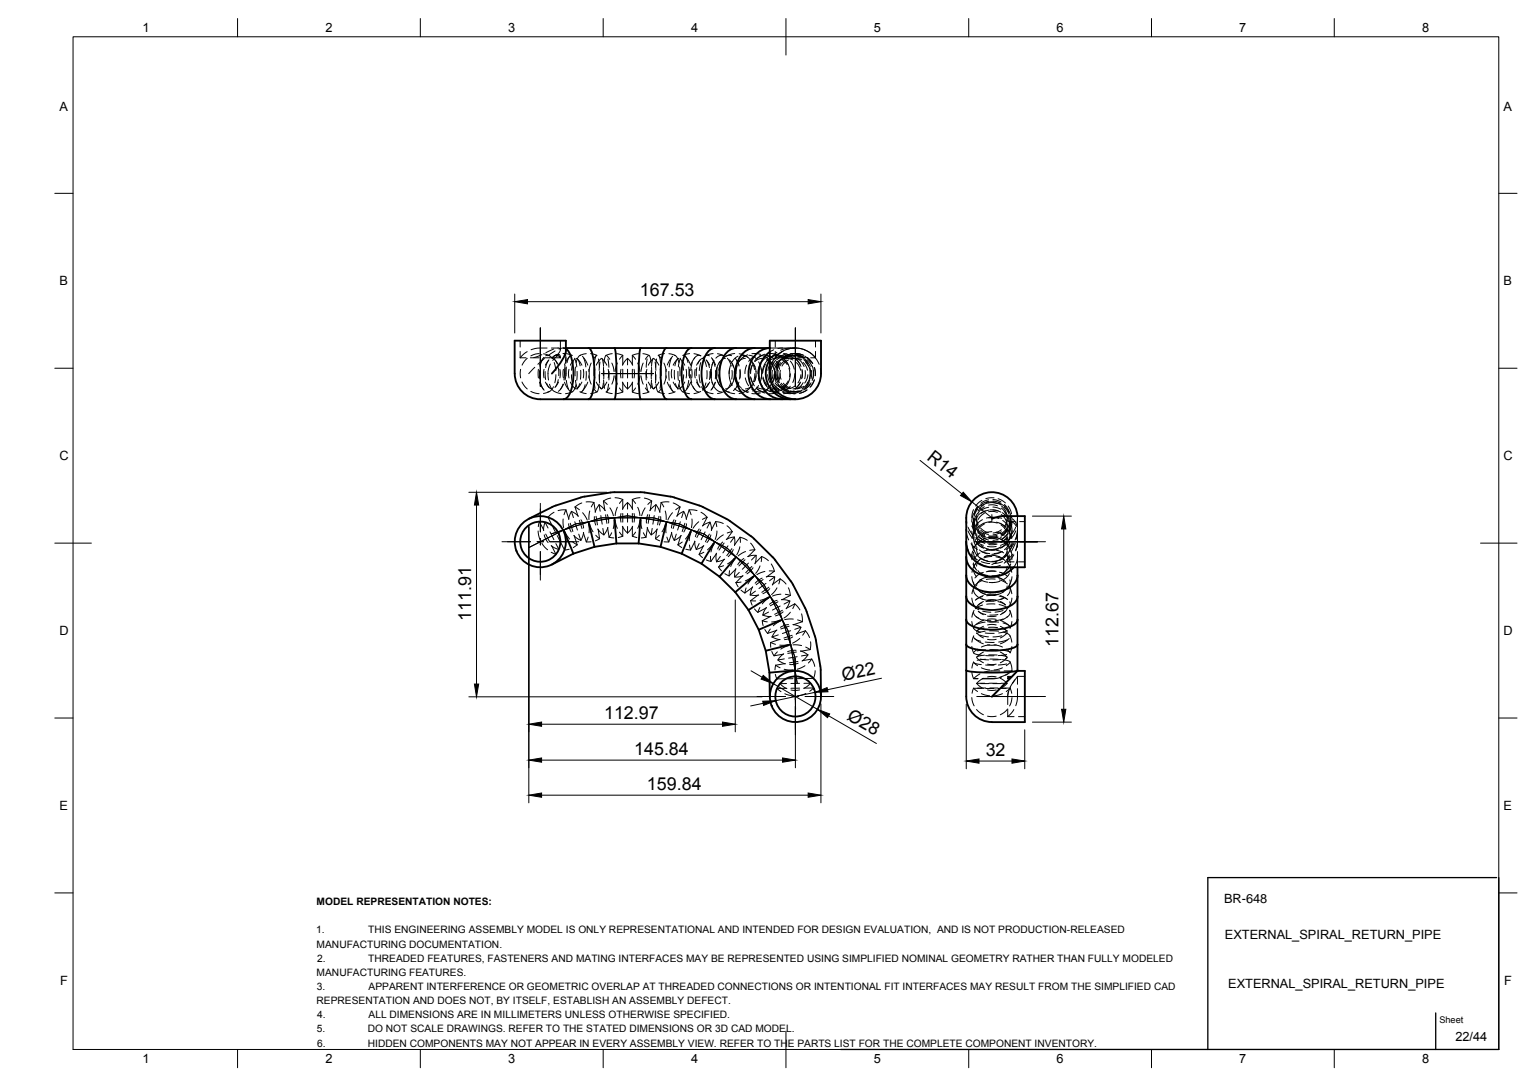
ISO-10303-21;
HEADER;
FILE_DESCRIPTION((''),'2;1');
FILE_NAME('EXTERNAL_SPIRAL_RETURN_PIPE.step','2026-10-01T22:05:39-07:00',(''),(''),'','','');
FILE_SCHEMA (('AUTOMOTIVE_DESIGN { 1 0 10303 214 3 1 1 }'));
ENDSEC;
DATA;
#10=MECHANICAL_DESIGN_GEOMETRIC_PRESENTATION_REPRESENTATION('',(#622),#24628);
#335=ELLIPSE('',#14693,1.97989898732233,1.4) ;
#336=ELLIPSE('',#14696,1.97989898732233,1.4) ;
#337=ELLIPSE('',#14700,1.40426046148572,1.4) ;
#338=ELLIPSE('',#14702,1.40426046148572,1.4) ;
#339=ELLIPSE('',#14708,1.40426046148572,1.4) ;
#340=ELLIPSE('',#14711,1.40426046148572,1.4) ;
#341=ELLIPSE('',#14714,1.40426046148572,1.4) ;
#342=ELLIPSE('',#14719,1.40426046148572,1.4) ;
#343=ELLIPSE('',#14724,1.40426046148572,1.4) ;
#344=ELLIPSE('',#14727,1.40426046148572,1.4) ;
#345=ELLIPSE('',#14730,1.40426046148572,1.4) ;
#346=ELLIPSE('',#14735,1.40426046148572,1.4) ;
#347=ELLIPSE('',#14740,1.40426046148572,1.4) ;
#348=ELLIPSE('',#14743,1.40426046148572,1.4) ;
#349=ELLIPSE('',#14746,1.40426046148572,1.4) ;
#350=ELLIPSE('',#14751,1.40426046148572,1.4) ;
#351=ELLIPSE('',#14756,1.97989898732233,1.4) ;
#352=ELLIPSE('',#14757,1.97989898732233,1.4) ;
#390=SPHERICAL_SURFACE('',#14496,1.1) ;
#391=SPHERICAL_SURFACE('',#14499,1.4) ;
#392=SPHERICAL_SURFACE('',#14501,1.1) ;
#393=SPHERICAL_SURFACE('',#14504,1.1) ;
#394=SPHERICAL_SURFACE('',#14506,1.1) ;
#395=SPHERICAL_SURFACE('',#14510,1.4) ;
#396=SPHERICAL_SURFACE('',#14511,1.4) ;
#397=SPHERICAL_SURFACE('',#14514,1.1) ;
#398=SPHERICAL_SURFACE('',#14517,1.4) ;
#399=SPHERICAL_SURFACE('',#14520,1.1) ;
#400=SPHERICAL_SURFACE('',#14524,1.4) ;
#401=SPHERICAL_SURFACE('',#14526,1.4) ;
#402=SPHERICAL_SURFACE('',#14528,1.1) ;
#403=SPHERICAL_SURFACE('',#14531,1.1) ;
#404=SPHERICAL_SURFACE('',#14533,1.4) ;
#405=SPHERICAL_SURFACE('',#14536,1.1) ;
#406=SPHERICAL_SURFACE('',#14539,1.4) ;
#407=SPHERICAL_SURFACE('',#14541,1.1) ;
#408=SPHERICAL_SURFACE('',#14545,1.4) ;
#409=SPHERICAL_SURFACE('',#14547,1.4) ;
#410=SPHERICAL_SURFACE('',#14549,1.1) ;
#411=SPHERICAL_SURFACE('',#14552,1.1) ;
#412=SPHERICAL_SURFACE('',#14554,1.4) ;
#413=SPHERICAL_SURFACE('',#14557,1.1) ;
#414=SPHERICAL_SURFACE('',#14560,1.4) ;
#415=SPHERICAL_SURFACE('',#14562,1.1) ;
#416=SPHERICAL_SURFACE('',#14566,1.4) ;
#417=SPHERICAL_SURFACE('',#14568,1.4) ;
#418=SPHERICAL_SURFACE('',#14570,1.1) ;
#419=SPHERICAL_SURFACE('',#14573,1.1) ;
#420=SPHERICAL_SURFACE('',#14575,1.4) ;
#421=SPHERICAL_SURFACE('',#14578,1.1) ;
#422=SPHERICAL_SURFACE('',#14581,1.4) ;
#423=SPHERICAL_SURFACE('',#14583,1.1) ;
#424=SPHERICAL_SURFACE('',#14587,1.4) ;
#425=SPHERICAL_SURFACE('',#14589,1.4) ;
#426=SPHERICAL_SURFACE('',#14590,1.1) ;
#427=SPHERICAL_SURFACE('',#14592,1.1) ;
#428=SPHERICAL_SURFACE('',#14593,1.4) ;
#429=SPHERICAL_SURFACE('',#14595,1.1) ;
#430=SPHERICAL_SURFACE('',#14598,1.4) ;
#431=SPHERICAL_SURFACE('',#14599,1.1) ;
#432=SPHERICAL_SURFACE('',#14603,1.4) ;
#433=SPHERICAL_SURFACE('',#14604,1.4) ;
#434=SPHERICAL_SURFACE('',#14605,1.1) ;
#435=SPHERICAL_SURFACE('',#14607,1.1) ;
#436=SPHERICAL_SURFACE('',#14608,1.4) ;
#437=SPHERICAL_SURFACE('',#14610,1.1) ;
#438=SPHERICAL_SURFACE('',#14615,1.4) ;
#439=SPHERICAL_SURFACE('',#14616,1.1) ;
#440=SPHERICAL_SURFACE('',#14622,1.4) ;
#441=SPHERICAL_SURFACE('',#14623,1.4) ;
#442=SPHERICAL_SURFACE('',#14624,1.1) ;
#443=SPHERICAL_SURFACE('',#14626,1.1) ;
#444=SPHERICAL_SURFACE('',#14627,1.4) ;
#445=SPHERICAL_SURFACE('',#14631,1.1) ;
#446=SPHERICAL_SURFACE('',#14632,1.1) ;
#447=SPHERICAL_SURFACE('',#14634,1.1) ;
#448=SPHERICAL_SURFACE('',#14635,1.4) ;
#449=SPHERICAL_SURFACE('',#14638,1.1) ;
#450=SPHERICAL_SURFACE('',#14641,1.4) ;
#451=SPHERICAL_SURFACE('',#14644,1.1) ;
#452=SPHERICAL_SURFACE('',#14650,1.4) ;
#453=SPHERICAL_SURFACE('',#14651,1.4) ;
#454=SPHERICAL_SURFACE('',#14656,1.4) ;
#455=SPHERICAL_SURFACE('',#14661,1.4) ;
#456=SPHERICAL_SURFACE('',#14666,1.4) ;
#457=SPHERICAL_SURFACE('',#14671,1.4) ;
#458=SPHERICAL_SURFACE('',#14676,1.4) ;
#459=SPHERICAL_SURFACE('',#14681,1.4) ;
#460=SPHERICAL_SURFACE('',#14684,1.4) ;
#461=SPHERICAL_SURFACE('',#14763,1.4) ;
#462=SPHERICAL_SURFACE('',#14764,1.4) ;
#463=SPHERICAL_SURFACE('',#14765,1.4) ;
#464=SPHERICAL_SURFACE('',#14766,1.4) ;
#465=SPHERICAL_SURFACE('',#14767,1.4) ;
#466=SPHERICAL_SURFACE('',#14768,1.4) ;
#467=SPHERICAL_SURFACE('',#14769,1.4) ;
#468=SPHERICAL_SURFACE('',#14773,1.4) ;
#469=SPHERICAL_SURFACE('',#14775,1.4) ;
#470=SPHERICAL_SURFACE('',#14776,1.1) ;
#471=SPHERICAL_SURFACE('',#14778,1.1) ;
#472=SPHERICAL_SURFACE('',#14779,1.1) ;
#473=SPHERICAL_SURFACE('',#14781,1.1) ;
#474=SPHERICAL_SURFACE('',#14782,1.1) ;
#475=SPHERICAL_SURFACE('',#14785,1.1) ;
#476=SPHERICAL_SURFACE('',#14787,1.1) ;
#477=SPHERICAL_SURFACE('',#14790,1.1) ;
#478=SPHERICAL_SURFACE('',#14792,1.1) ;
#479=SPHERICAL_SURFACE('',#14795,1.1) ;
#480=SPHERICAL_SURFACE('',#14797,1.1) ;
#481=SPHERICAL_SURFACE('',#14800,1.1) ;
#487=ORIENTED_CLOSED_SHELL('',*,#13133,.F.) ;
#488=ORIENTED_CLOSED_SHELL('',*,#13134,.F.) ;
#489=ORIENTED_CLOSED_SHELL('',*,#13135,.F.) ;
#490=ORIENTED_CLOSED_SHELL('',*,#13136,.F.) ;
#491=ORIENTED_CLOSED_SHELL('',*,#13137,.F.) ;
#492=ORIENTED_CLOSED_SHELL('',*,#13138,.F.) ;
#493=ORIENTED_CLOSED_SHELL('',*,#13139,.F.) ;
#494=ORIENTED_CLOSED_SHELL('',*,#13140,.F.) ;
#495=ORIENTED_CLOSED_SHELL('',*,#13141,.F.) ;
#496=ORIENTED_CLOSED_SHELL('',*,#13142,.F.) ;
#497=ORIENTED_CLOSED_SHELL('',*,#13143,.F.) ;
#498=ORIENTED_CLOSED_SHELL('',*,#13144,.F.) ;
#499=ORIENTED_CLOSED_SHELL('',*,#13145,.F.) ;
#500=ORIENTED_CLOSED_SHELL('',*,#13146,.F.) ;
#501=ORIENTED_CLOSED_SHELL('',*,#13147,.F.) ;
#502=ORIENTED_CLOSED_SHELL('',*,#13148,.F.) ;
#503=ORIENTED_CLOSED_SHELL('',*,#13149,.F.) ;
#504=ORIENTED_CLOSED_SHELL('',*,#13150,.F.) ;
#505=ORIENTED_CLOSED_SHELL('',*,#13151,.F.) ;
#506=ORIENTED_CLOSED_SHELL('',*,#13152,.F.) ;
#507=ORIENTED_CLOSED_SHELL('',*,#13153,.F.) ;
#508=ORIENTED_CLOSED_SHELL('',*,#13154,.F.) ;
#509=ORIENTED_CLOSED_SHELL('',*,#13155,.F.) ;
#510=ORIENTED_CLOSED_SHELL('',*,#13156,.F.) ;
#511=ORIENTED_CLOSED_SHELL('',*,#13157,.F.) ;
#512=ORIENTED_CLOSED_SHELL('',*,#13159,.F.) ;
#513=ORIENTED_CLOSED_SHELL('',*,#13160,.F.) ;
#514=ORIENTED_CLOSED_SHELL('',*,#13161,.F.) ;
#515=ORIENTED_CLOSED_SHELL('',*,#13162,.F.) ;
#516=ORIENTED_CLOSED_SHELL('',*,#13163,.F.) ;
#517=ORIENTED_CLOSED_SHELL('',*,#13164,.F.) ;
#520=BREP_WITH_VOIDS('EXTERNAL_SPIRAL_RETURN_PIPE',#13158,(#487,#488,#489,
#490,#491,#492,#493,#494,#495,#496,#497,#498,#499,#500,#501,#502,#503,#504,
#505,#506,#507,#508,#509,#510,#511,#512,#513,#514,#515,#516,#517)) ;
#538=SHAPE_REPRESENTATION_RELATIONSHIP('SRR','None',#24810,#580) ;
#580=ADVANCED_BREP_SHAPE_REPRESENTATION('',(#520),#24600) ;
#622=STYLED_ITEM('',(#25037),#520) ;
#857=FACE_BOUND('',#4291,.T.) ;
#858=FACE_BOUND('',#4298,.T.) ;
#859=FACE_BOUND('',#4301,.T.) ;
#860=FACE_BOUND('',#4315,.T.) ;
#861=FACE_BOUND('',#4329,.T.) ;
#862=FACE_BOUND('',#4348,.T.) ;
#956=B_SPLINE_CURVE_WITH_KNOTS('',3,(#21637,#21638,#21639,#21640,#21641,
#21642,#21643,#21644,#21645,#21646,#21647,#21648,#21649,#21650),
 .UNSPECIFIED.,.F.,.F.,(4,2,2,2,2,2,4),(1.10605212017019,1.19682866015767,
1.42236457431749,1.64790048847731,1.87343640263713,2.09897231679695,2.18974885678443),
 .UNSPECIFIED.) ;
#957=B_SPLINE_CURVE_WITH_KNOTS('',3,(#21663,#21664,#21665,#21666,#21667,
#21668,#21669,#21670,#21671,#21672,#21673,#21674,#21675,#21676,#21677,#21678,
#21679,#21680,#21681,#21682,#21683,#21684,#21685,#21686,#21687,#21688),
 .UNSPECIFIED.,.F.,.F.,(4,2,2,2,2,2,2,2,2,2,2,2,4),(1.20535125846133,1.58564147586808,
1.96593169327483,2.13946869190595,2.31300569053706,2.5849459608724,2.85688623120774,
3.12882650154308,3.40076677187842,3.57430377050953,3.74784076914065,4.1281309865474,
4.50842120395415),.UNSPECIFIED.) ;
#958=B_SPLINE_CURVE_WITH_KNOTS('',3,(#21860,#21861,#21862,#21863,#21864,
#21865,#21866,#21867,#21868,#21869),.UNSPECIFIED.,.F.,.F.,(4,2,2,2,4),(2.19179053945309,
2.41386787047132,2.73532606912548,3.05678426777964,3.27886159879787),
 .UNSPECIFIED.) ;
#959=B_SPLINE_CURVE_WITH_KNOTS('',3,(#21899,#21900,#21901,#21902,#21903,
#21904,#21905,#21906,#21907,#21908,#21909,#21910,#21911,#21912,#21913,#21914,
#21915,#21916,#21917,#21918,#21919,#21920),.UNSPECIFIED.,.F.,.F.,(4,2,2,
2,2,2,2,2,2,2,4),(1.21055307378235,1.62541412185573,2.04027516992911,2.46215750524915,
2.67309867290916,2.88403984056918,3.0949810082292,3.30592217588921,3.72780451120925,
4.14266555928263,4.557526607356),.UNSPECIFIED.) ;
#960=B_SPLINE_CURVE_WITH_KNOTS('',3,(#21996,#21997,#21998,#21999,#22000,
#22001),.UNSPECIFIED.,.F.,.F.,(4,2,4),(3.13976161696689,3.31479971489035,
3.53911083723209),.UNSPECIFIED.) ;
#961=B_SPLINE_CURVE_WITH_KNOTS('',3,(#22002,#22003,#22004,#22005,#22006,
#22007,#22008,#22009,#22010,#22011,#22012,#22013,#22014,#22015,#22016,#22017,
#22018,#22019,#22020,#22021,#22022,#22023,#22024,#22025),.UNSPECIFIED.,
 .F.,.F.,(4,2,2,2,2,2,2,2,2,2,2,4),(0.,0.224311122341738,0.448622244683475,
0.897244489366951,1.3333999539915,1.55147768630377,1.76955541861604,1.98763315092831,
2.20571088324059,2.64186634786513,3.09048859254861,3.13976161696689),
 .UNSPECIFIED.) ;
#962=B_SPLINE_CURVE_WITH_KNOTS('',3,(#22053,#22054,#22055,#22056,#22057,
#22058,#22059,#22060,#22061,#22062,#22063,#22064,#22065,#22066),
 .UNSPECIFIED.,.F.,.F.,(4,2,2,2,2,2,4),(-3.53911083723208,-3.31479971489035,
-3.09048859254861,-2.64186634786513,-2.20571088324059,-1.98763315092831,
-1.87498686215861),.UNSPECIFIED.) ;
#963=B_SPLINE_CURVE_WITH_KNOTS('',3,(#22068,#22069,#22070,#22071,#22072,
#22073,#22074,#22075,#22076,#22077,#22078,#22079,#22080,#22081,#22082,#22083),
 .UNSPECIFIED.,.F.,.F.,(4,2,2,2,2,2,2,4),(-1.87498686215861,-1.76955541861604,
-1.55147768630377,-1.3333999539915,-0.89724448936695,-0.448622244683476,
-0.224311122341738,0.),.UNSPECIFIED.) ;
#1388=LINE('',#21995,#2224) ;
#1389=LINE('',#22030,#2225) ;
#1390=LINE('',#22043,#2226) ;
#1391=LINE('',#22088,#2227) ;
#1392=LINE('',#22092,#2228) ;
#1393=LINE('',#22096,#2229) ;
#1394=LINE('',#22106,#2230) ;
#1395=LINE('',#22116,#2231) ;
#1396=LINE('',#22120,#2232) ;
#1397=LINE('',#22124,#2233) ;
#1398=LINE('',#22134,#2234) ;
#1399=LINE('',#22144,#2235) ;
#1400=LINE('',#22148,#2236) ;
#1401=LINE('',#22152,#2237) ;
#1402=LINE('',#22162,#2238) ;
#1403=LINE('',#22172,#2239) ;
#1404=LINE('',#22180,#2240) ;
#1405=LINE('',#22194,#2241) ;
#2224=VECTOR('',#17855,1.1) ;
#2225=VECTOR('',#17860,1.4) ;
#2226=VECTOR('',#17875,1.4) ;
#2227=VECTOR('',#17892,1.4) ;
#2228=VECTOR('',#17899,1.4) ;
#2229=VECTOR('',#17904,1.4) ;
#2230=VECTOR('',#17915,1.4) ;
#2231=VECTOR('',#17928,1.4) ;
#2232=VECTOR('',#17935,1.4) ;
#2233=VECTOR('',#17940,1.4) ;
#2234=VECTOR('',#17951,1.4) ;
#2235=VECTOR('',#17964,1.4) ;
#2236=VECTOR('',#17971,1.4) ;
#2237=VECTOR('',#17976,1.4) ;
#2238=VECTOR('',#17987,1.4) ;
#2239=VECTOR('',#18000,1.4) ;
#2240=VECTOR('',#18011,1.4) ;
#2241=VECTOR('',#18036,1.1) ;
#2844=CYLINDRICAL_SURFACE('',#14508,1.1) ;
#2845=CYLINDRICAL_SURFACE('',#14519,1.4) ;
#2846=CYLINDRICAL_SURFACE('',#14630,1.1) ;
#2847=CYLINDRICAL_SURFACE('',#14649,1.4) ;
#2848=CYLINDRICAL_SURFACE('',#14689,1.1) ;
#2849=CYLINDRICAL_SURFACE('',#14691,1.4) ;
#2850=CYLINDRICAL_SURFACE('',#14699,1.4) ;
#2851=CYLINDRICAL_SURFACE('',#14704,1.4) ;
#2852=CYLINDRICAL_SURFACE('',#14706,1.4) ;
#2853=CYLINDRICAL_SURFACE('',#14710,1.4) ;
#2854=CYLINDRICAL_SURFACE('',#14712,1.4) ;
#2855=CYLINDRICAL_SURFACE('',#14716,1.4) ;
#2856=CYLINDRICAL_SURFACE('',#14722,1.4) ;
#2857=CYLINDRICAL_SURFACE('',#14726,1.4) ;
#2858=CYLINDRICAL_SURFACE('',#14728,1.4) ;
#2859=CYLINDRICAL_SURFACE('',#14732,1.4) ;
#2860=CYLINDRICAL_SURFACE('',#14738,1.4) ;
#2861=CYLINDRICAL_SURFACE('',#14742,1.4) ;
#2862=CYLINDRICAL_SURFACE('',#14744,1.4) ;
#2863=CYLINDRICAL_SURFACE('',#14748,1.4) ;
#2864=CYLINDRICAL_SURFACE('',#14754,1.4) ;
#2865=CYLINDRICAL_SURFACE('',#14759,1.4) ;
#2866=CYLINDRICAL_SURFACE('',#14760,1.4) ;
#2867=CYLINDRICAL_SURFACE('',#14771,1.1) ;
#3309=FACE_OUTER_BOUND('',#4247,.T.) ;
#3310=FACE_OUTER_BOUND('',#4248,.T.) ;
#3311=FACE_OUTER_BOUND('',#4249,.T.) ;
#3312=FACE_OUTER_BOUND('',#4250,.T.) ;
#3313=FACE_OUTER_BOUND('',#4251,.T.) ;
#3314=FACE_OUTER_BOUND('',#4252,.T.) ;
#3315=FACE_OUTER_BOUND('',#4253,.T.) ;
#3316=FACE_OUTER_BOUND('',#4254,.T.) ;
#3317=FACE_OUTER_BOUND('',#4255,.T.) ;
#3318=FACE_OUTER_BOUND('',#4256,.T.) ;
#3319=FACE_OUTER_BOUND('',#4257,.T.) ;
#3320=FACE_OUTER_BOUND('',#4258,.T.) ;
#3321=FACE_OUTER_BOUND('',#4259,.T.) ;
#3322=FACE_OUTER_BOUND('',#4260,.T.) ;
#3323=FACE_OUTER_BOUND('',#4261,.T.) ;
#3324=FACE_OUTER_BOUND('',#4262,.T.) ;
#3325=FACE_OUTER_BOUND('',#4263,.T.) ;
#3326=FACE_OUTER_BOUND('',#4264,.T.) ;
#3327=FACE_OUTER_BOUND('',#4265,.T.) ;
#3328=FACE_OUTER_BOUND('',#4266,.T.) ;
#3329=FACE_OUTER_BOUND('',#4267,.T.) ;
#3330=FACE_OUTER_BOUND('',#4268,.T.) ;
#3331=FACE_OUTER_BOUND('',#4269,.T.) ;
#3332=FACE_OUTER_BOUND('',#4270,.T.) ;
#3333=FACE_OUTER_BOUND('',#4271,.T.) ;
#3334=FACE_OUTER_BOUND('',#4272,.T.) ;
#3335=FACE_OUTER_BOUND('',#4273,.T.) ;
#3336=FACE_OUTER_BOUND('',#4274,.T.) ;
#3337=FACE_OUTER_BOUND('',#4275,.T.) ;
#3338=FACE_OUTER_BOUND('',#4276,.T.) ;
#3339=FACE_OUTER_BOUND('',#4277,.T.) ;
#3340=FACE_OUTER_BOUND('',#4278,.T.) ;
#3341=FACE_OUTER_BOUND('',#4279,.T.) ;
#3342=FACE_OUTER_BOUND('',#4280,.T.) ;
#3343=FACE_OUTER_BOUND('',#4281,.T.) ;
#3344=FACE_OUTER_BOUND('',#4282,.T.) ;
#3345=FACE_OUTER_BOUND('',#4283,.T.) ;
#3346=FACE_OUTER_BOUND('',#4284,.T.) ;
#3347=FACE_OUTER_BOUND('',#4285,.T.) ;
#3348=FACE_OUTER_BOUND('',#4286,.T.) ;
#3349=FACE_OUTER_BOUND('',#4287,.T.) ;
#3350=FACE_OUTER_BOUND('',#4288,.T.) ;
#3351=FACE_OUTER_BOUND('',#4289,.T.) ;
#3352=FACE_OUTER_BOUND('',#4290,.T.) ;
#3353=FACE_OUTER_BOUND('',#4292,.T.) ;
#3354=FACE_OUTER_BOUND('',#4293,.T.) ;
#3355=FACE_OUTER_BOUND('',#4294,.T.) ;
#3356=FACE_OUTER_BOUND('',#4295,.T.) ;
#3357=FACE_OUTER_BOUND('',#4296,.T.) ;
#3358=FACE_OUTER_BOUND('',#4297,.T.) ;
#3359=FACE_OUTER_BOUND('',#4299,.T.) ;
#3360=FACE_OUTER_BOUND('',#4300,.T.) ;
#3361=FACE_OUTER_BOUND('',#4302,.T.) ;
#3362=FACE_OUTER_BOUND('',#4303,.T.) ;
#3363=FACE_OUTER_BOUND('',#4304,.T.) ;
#3364=FACE_OUTER_BOUND('',#4305,.T.) ;
#3365=FACE_OUTER_BOUND('',#4306,.T.) ;
#3366=FACE_OUTER_BOUND('',#4307,.T.) ;
#3367=FACE_OUTER_BOUND('',#4308,.T.) ;
#3368=FACE_OUTER_BOUND('',#4309,.T.) ;
#3369=FACE_OUTER_BOUND('',#4310,.T.) ;
#3370=FACE_OUTER_BOUND('',#4311,.T.) ;
#3371=FACE_OUTER_BOUND('',#4312,.T.) ;
#3372=FACE_OUTER_BOUND('',#4313,.T.) ;
#3373=FACE_OUTER_BOUND('',#4314,.T.) ;
#3374=FACE_OUTER_BOUND('',#4316,.T.) ;
#3375=FACE_OUTER_BOUND('',#4317,.T.) ;
#3376=FACE_OUTER_BOUND('',#4318,.T.) ;
#3377=FACE_OUTER_BOUND('',#4319,.T.) ;
#3378=FACE_OUTER_BOUND('',#4320,.T.) ;
#3379=FACE_OUTER_BOUND('',#4321,.T.) ;
#3380=FACE_OUTER_BOUND('',#4322,.T.) ;
#3381=FACE_OUTER_BOUND('',#4323,.T.) ;
#3382=FACE_OUTER_BOUND('',#4324,.T.) ;
#3383=FACE_OUTER_BOUND('',#4325,.T.) ;
#3384=FACE_OUTER_BOUND('',#4326,.T.) ;
#3385=FACE_OUTER_BOUND('',#4327,.T.) ;
#3386=FACE_OUTER_BOUND('',#4328,.T.) ;
#3387=FACE_OUTER_BOUND('',#4330,.T.) ;
#3388=FACE_OUTER_BOUND('',#4331,.T.) ;
#3389=FACE_OUTER_BOUND('',#4332,.T.) ;
#3390=FACE_OUTER_BOUND('',#4333,.T.) ;
#3391=FACE_OUTER_BOUND('',#4334,.T.) ;
#3392=FACE_OUTER_BOUND('',#4335,.T.) ;
#3393=FACE_OUTER_BOUND('',#4336,.T.) ;
#3394=FACE_OUTER_BOUND('',#4337,.T.) ;
#3395=FACE_OUTER_BOUND('',#4338,.T.) ;
#3396=FACE_OUTER_BOUND('',#4339,.T.) ;
#3397=FACE_OUTER_BOUND('',#4340,.T.) ;
#3398=FACE_OUTER_BOUND('',#4341,.T.) ;
#3399=FACE_OUTER_BOUND('',#4342,.T.) ;
#3400=FACE_OUTER_BOUND('',#4343,.T.) ;
#3401=FACE_OUTER_BOUND('',#4344,.T.) ;
#3402=FACE_OUTER_BOUND('',#4345,.T.) ;
#3403=FACE_OUTER_BOUND('',#4346,.T.) ;
#3404=FACE_OUTER_BOUND('',#4347,.T.) ;
#3405=FACE_OUTER_BOUND('',#4349,.T.) ;
#3406=FACE_OUTER_BOUND('',#4350,.T.) ;
#3407=FACE_OUTER_BOUND('',#4351,.T.) ;
#3408=FACE_OUTER_BOUND('',#4352,.T.) ;
#3409=FACE_OUTER_BOUND('',#4353,.T.) ;
#3410=FACE_OUTER_BOUND('',#4354,.T.) ;
#3411=FACE_OUTER_BOUND('',#4355,.T.) ;
#3412=FACE_OUTER_BOUND('',#4356,.T.) ;
#3413=FACE_OUTER_BOUND('',#4357,.T.) ;
#3414=FACE_OUTER_BOUND('',#4358,.T.) ;
#3415=FACE_OUTER_BOUND('',#4359,.T.) ;
#3416=FACE_OUTER_BOUND('',#4360,.T.) ;
#3417=FACE_OUTER_BOUND('',#4361,.T.) ;
#3418=FACE_OUTER_BOUND('',#4362,.T.) ;
#3419=FACE_OUTER_BOUND('',#4363,.T.) ;
#3420=FACE_OUTER_BOUND('',#4364,.T.) ;
#3421=FACE_OUTER_BOUND('',#4365,.T.) ;
#3422=FACE_OUTER_BOUND('',#4366,.T.) ;
#3423=FACE_OUTER_BOUND('',#4367,.T.) ;
#3424=FACE_OUTER_BOUND('',#4368,.T.) ;
#3425=FACE_OUTER_BOUND('',#4369,.T.) ;
#3426=FACE_OUTER_BOUND('',#4370,.T.) ;
#4247=EDGE_LOOP('',(#10205,#10206,#10207)) ;
#4248=EDGE_LOOP('',(#10208,#10209,#10210)) ;
#4249=EDGE_LOOP('',(#10211,#10212,#10213)) ;
#4250=EDGE_LOOP('',(#10214,#10215,#10216)) ;
#4251=EDGE_LOOP('',(#10217,#10218)) ;
#4252=EDGE_LOOP('',(#10219,#10220)) ;
#4253=EDGE_LOOP('',(#10221,#10222)) ;
#4254=EDGE_LOOP('',(#10223,#10224,#10225)) ;
#4255=EDGE_LOOP('',(#10226,#10227,#10228,#10229,#10230)) ;
#4256=EDGE_LOOP('',(#10231,#10232)) ;
#4257=EDGE_LOOP('',(#10233,#10234)) ;
#4258=EDGE_LOOP('',(#10235,#10236,#10237,#10238)) ;
#4259=EDGE_LOOP('',(#10239,#10240,#10241)) ;
#4260=EDGE_LOOP('',(#10242,#10243,#10244)) ;
#4261=EDGE_LOOP('',(#10245,#10246,#10247)) ;
#4262=EDGE_LOOP('',(#10248,#10249,#10250)) ;
#4263=EDGE_LOOP('',(#10251,#10252,#10253)) ;
#4264=EDGE_LOOP('',(#10254,#10255,#10256,#10257)) ;
#4265=EDGE_LOOP('',(#10258,#10259,#10260)) ;
#4266=EDGE_LOOP('',(#10261,#10262,#10263,#10264)) ;
#4267=EDGE_LOOP('',(#10265,#10266,#10267)) ;
#4268=EDGE_LOOP('',(#10268,#10269,#10270)) ;
#4269=EDGE_LOOP('',(#10271,#10272,#10273)) ;
#4270=EDGE_LOOP('',(#10274,#10275,#10276)) ;
#4271=EDGE_LOOP('',(#10277,#10278,#10279)) ;
#4272=EDGE_LOOP('',(#10280,#10281,#10282,#10283)) ;
#4273=EDGE_LOOP('',(#10284,#10285,#10286)) ;
#4274=EDGE_LOOP('',(#10287,#10288,#10289,#10290)) ;
#4275=EDGE_LOOP('',(#10291,#10292,#10293)) ;
#4276=EDGE_LOOP('',(#10294,#10295,#10296)) ;
#4277=EDGE_LOOP('',(#10297,#10298,#10299)) ;
#4278=EDGE_LOOP('',(#10300,#10301,#10302)) ;
#4279=EDGE_LOOP('',(#10303,#10304,#10305)) ;
#4280=EDGE_LOOP('',(#10306,#10307,#10308,#10309)) ;
#4281=EDGE_LOOP('',(#10310,#10311,#10312)) ;
#4282=EDGE_LOOP('',(#10313,#10314,#10315,#10316)) ;
#4283=EDGE_LOOP('',(#10317,#10318,#10319)) ;
#4284=EDGE_LOOP('',(#10320)) ;
#4285=EDGE_LOOP('',(#10321)) ;
#4286=EDGE_LOOP('',(#10322)) ;
#4287=EDGE_LOOP('',(#10323)) ;
#4288=EDGE_LOOP('',(#10324,#10325,#10326,#10327)) ;
#4289=EDGE_LOOP('',(#10328)) ;
#4290=EDGE_LOOP('',(#10329,#10330,#10331)) ;
#4291=EDGE_LOOP('',(#10332)) ;
#4292=EDGE_LOOP('',(#10333)) ;
#4293=EDGE_LOOP('',(#10334)) ;
#4294=EDGE_LOOP('',(#10335)) ;
#4295=EDGE_LOOP('',(#10336)) ;
#4296=EDGE_LOOP('',(#10337)) ;
#4297=EDGE_LOOP('',(#10338,#10339,#10340,#10341,#10342,#10343)) ;
#4298=EDGE_LOOP('',(#10344)) ;
#4299=EDGE_LOOP('',(#10345,#10346)) ;
#4300=EDGE_LOOP('',(#10347,#10348,#10349,#10350,#10351,#10352)) ;
#4301=EDGE_LOOP('',(#10353)) ;
#4302=EDGE_LOOP('',(#10354,#10355)) ;
#4303=EDGE_LOOP('',(#10356)) ;
#4304=EDGE_LOOP('',(#10357)) ;
#4305=EDGE_LOOP('',(#10358)) ;
#4306=EDGE_LOOP('',(#10359,#10360)) ;
#4307=EDGE_LOOP('',(#10361,#10362)) ;
#4308=EDGE_LOOP('',(#10363,#10364)) ;
#4309=EDGE_LOOP('',(#10365)) ;
#4310=EDGE_LOOP('',(#10366)) ;
#4311=EDGE_LOOP('',(#10367,#10368)) ;
#4312=EDGE_LOOP('',(#10369,#10370,#10371,#10372,#10373,#10374)) ;
#4313=EDGE_LOOP('',(#10375,#10376)) ;
#4314=EDGE_LOOP('',(#10377,#10378,#10379,#10380,#10381,#10382)) ;
#4315=EDGE_LOOP('',(#10383,#10384)) ;
#4316=EDGE_LOOP('',(#10385,#10386)) ;
#4317=EDGE_LOOP('',(#10387,#10388)) ;
#4318=EDGE_LOOP('',(#10389,#10390,#10391,#10392)) ;
#4319=EDGE_LOOP('',(#10393,#10394,#10395,#10396)) ;
#4320=EDGE_LOOP('',(#10397,#10398,#10399,#10400)) ;
#4321=EDGE_LOOP('',(#10401,#10402,#10403,#10404)) ;
#4322=EDGE_LOOP('',(#10405,#10406,#10407,#10408)) ;
#4323=EDGE_LOOP('',(#10409,#10410,#10411,#10412)) ;
#4324=EDGE_LOOP('',(#10413,#10414)) ;
#4325=EDGE_LOOP('',(#10415,#10416,#10417,#10418,#10419)) ;
#4326=EDGE_LOOP('',(#10420,#10421,#10422,#10423,#10424,#10425)) ;
#4327=EDGE_LOOP('',(#10426,#10427,#10428,#10429,#10430,#10431,#10432)) ;
#4328=EDGE_LOOP('',(#10433)) ;
#4329=EDGE_LOOP('',(#10434)) ;
#4330=EDGE_LOOP('',(#10435,#10436,#10437,#10438,#10439,#10440,#10441,#10442)) ;
#4331=EDGE_LOOP('',(#10443,#10444,#10445)) ;
#4332=EDGE_LOOP('',(#10446,#10447,#10448,#10449,#10450,#10451,#10452,#10453,
#10454)) ;
#4333=EDGE_LOOP('',(#10455,#10456,#10457,#10458,#10459,#10460,#10461,#10462)) ;
#4334=EDGE_LOOP('',(#10463,#10464,#10465,#10466,#10467,#10468,#10469,#10470)) ;
#4335=EDGE_LOOP('',(#10471,#10472,#10473,#10474,#10475,#10476,#10477,#10478)) ;
#4336=EDGE_LOOP('',(#10479,#10480,#10481,#10482,#10483,#10484,#10485,#10486)) ;
#4337=EDGE_LOOP('',(#10487,#10488,#10489,#10490,#10491,#10492,#10493,#10494)) ;
#4338=EDGE_LOOP('',(#10495,#10496,#10497,#10498,#10499,#10500,#10501,#10502)) ;
#4339=EDGE_LOOP('',(#10503,#10504,#10505,#10506,#10507,#10508,#10509,#10510)) ;
#4340=EDGE_LOOP('',(#10511,#10512,#10513,#10514,#10515,#10516,#10517,#10518)) ;
#4341=EDGE_LOOP('',(#10519,#10520,#10521,#10522,#10523,#10524,#10525,#10526)) ;
#4342=EDGE_LOOP('',(#10527,#10528,#10529,#10530,#10531,#10532,#10533,#10534)) ;
#4343=EDGE_LOOP('',(#10535,#10536,#10537,#10538,#10539,#10540,#10541,#10542)) ;
#4344=EDGE_LOOP('',(#10543,#10544,#10545,#10546,#10547,#10548,#10549,#10550,
#10551)) ;
#4345=EDGE_LOOP('',(#10552,#10553,#10554)) ;
#4346=EDGE_LOOP('',(#10555,#10556,#10557,#10558,#10559,#10560)) ;
#4347=EDGE_LOOP('',(#10561)) ;
#4348=EDGE_LOOP('',(#10562)) ;
#4349=EDGE_LOOP('',(#10563,#10564,#10565,#10566)) ;
#4350=EDGE_LOOP('',(#10567,#10568,#10569,#10570)) ;
#4351=EDGE_LOOP('',(#10571,#10572,#10573,#10574)) ;
#4352=EDGE_LOOP('',(#10575,#10576,#10577,#10578)) ;
#4353=EDGE_LOOP('',(#10579,#10580,#10581,#10582)) ;
#4354=EDGE_LOOP('',(#10583,#10584,#10585,#10586)) ;
#4355=EDGE_LOOP('',(#10587,#10588,#10589,#10590,#10591)) ;
#4356=EDGE_LOOP('',(#10592,#10593,#10594,#10595,#10596,#10597)) ;
#4357=EDGE_LOOP('',(#10598,#10599,#10600,#10601,#10602)) ;
#4358=EDGE_LOOP('',(#10603,#10604)) ;
#4359=EDGE_LOOP('',(#10605)) ;
#4360=EDGE_LOOP('',(#10606)) ;
#4361=EDGE_LOOP('',(#10607)) ;
#4362=EDGE_LOOP('',(#10608)) ;
#4363=EDGE_LOOP('',(#10609,#10610,#10611)) ;
#4364=EDGE_LOOP('',(#10612,#10613,#10614)) ;
#4365=EDGE_LOOP('',(#10615,#10616,#10617)) ;
#4366=EDGE_LOOP('',(#10618,#10619,#10620)) ;
#4367=EDGE_LOOP('',(#10621,#10622,#10623)) ;
#4368=EDGE_LOOP('',(#10624,#10625,#10626)) ;
#4369=EDGE_LOOP('',(#10627,#10628,#10629)) ;
#4370=EDGE_LOOP('',(#10630,#10631,#10632)) ;
#5160=CIRCLE('',#14497,1.00181590545205) ;
#5161=CIRCLE('',#14498,1.1) ;
#5162=CIRCLE('',#14500,1.4) ;
#5163=CIRCLE('',#14502,0.834979872033575) ;
#5164=CIRCLE('',#14503,1.1) ;
#5165=CIRCLE('',#14505,1.1) ;
#5166=CIRCLE('',#14507,1.00181590545205) ;
#5167=CIRCLE('',#14509,1.1) ;
#5168=CIRCLE('',#14512,1.00181590545205) ;
#5169=CIRCLE('',#14513,1.4) ;
#5170=CIRCLE('',#14515,1.1) ;
#5171=CIRCLE('',#14516,1.00181590545205) ;
#5172=CIRCLE('',#14518,1.4) ;
#5173=CIRCLE('',#14521,1.00181590545205) ;
#5174=CIRCLE('',#14522,1.1) ;
#5175=CIRCLE('',#14523,1.00181590545205) ;
#5176=CIRCLE('',#14525,1.4) ;
#5177=CIRCLE('',#14527,1.4) ;
#5178=CIRCLE('',#14529,0.834979872033575) ;
#5179=CIRCLE('',#14530,1.1) ;
#5180=CIRCLE('',#14532,1.1) ;
#5181=CIRCLE('',#14534,1.00181590545205) ;
#5182=CIRCLE('',#14535,1.4) ;
#5183=CIRCLE('',#14537,1.1) ;
#5184=CIRCLE('',#14538,1.00181590545205) ;
#5185=CIRCLE('',#14540,1.4) ;
#5186=CIRCLE('',#14542,1.00181590545205) ;
#5187=CIRCLE('',#14543,1.1) ;
#5188=CIRCLE('',#14544,1.00181590545205) ;
#5189=CIRCLE('',#14546,1.4) ;
#5190=CIRCLE('',#14548,1.4) ;
#5191=CIRCLE('',#14550,0.834979872033577) ;
#5192=CIRCLE('',#14551,1.1) ;
#5193=CIRCLE('',#14553,1.1) ;
#5194=CIRCLE('',#14555,1.00181590545205) ;
#5195=CIRCLE('',#14556,1.4) ;
#5196=CIRCLE('',#14558,1.1) ;
#5197=CIRCLE('',#14559,1.00181590545205) ;
#5198=CIRCLE('',#14561,1.4) ;
#5199=CIRCLE('',#14563,1.00181590545205) ;
#5200=CIRCLE('',#14564,1.1) ;
#5201=CIRCLE('',#14565,1.00181590545205) ;
#5202=CIRCLE('',#14567,1.4) ;
#5203=CIRCLE('',#14569,1.4) ;
#5204=CIRCLE('',#14571,0.834979872033573) ;
#5205=CIRCLE('',#14572,1.1) ;
#5206=CIRCLE('',#14574,1.1) ;
#5207=CIRCLE('',#14576,1.00181590545205) ;
#5208=CIRCLE('',#14577,1.4) ;
#5209=CIRCLE('',#14579,1.1) ;
#5210=CIRCLE('',#14580,1.00181590545205) ;
#5211=CIRCLE('',#14582,1.4) ;
#5212=CIRCLE('',#14584,1.00181590545205) ;
#5213=CIRCLE('',#14585,1.1) ;
#5214=CIRCLE('',#14586,1.00181590545205) ;
#5215=CIRCLE('',#14588,1.4) ;
#5216=CIRCLE('',#14591,0.834979872033577) ;
#5217=CIRCLE('',#14594,1.00181590545205) ;
#5218=CIRCLE('',#14596,1.1) ;
#5219=CIRCLE('',#14597,1.00181590545205) ;
#5220=CIRCLE('',#14600,1.00181590545205) ;
#5221=CIRCLE('',#14601,1.1) ;
#5222=CIRCLE('',#14602,1.00181590545205) ;
#5223=CIRCLE('',#14606,0.834979872033575) ;
#5224=CIRCLE('',#14609,1.00181590545205) ;
#5225=CIRCLE('',#14611,1.00181590545205) ;
#5226=CIRCLE('',#14612,1.1) ;
#5227=CIRCLE('',#14613,1.00181590545205) ;
#5228=CIRCLE('',#14614,1.1) ;
#5229=CIRCLE('',#14617,1.00181590545205) ;
#5230=CIRCLE('',#14618,1.1) ;
#5231=CIRCLE('',#14619,1.00181590545205) ;
#5232=CIRCLE('',#14620,1.1) ;
#5233=CIRCLE('',#14621,1.00181590545205) ;
#5234=CIRCLE('',#14625,0.834979872033575) ;
#5235=CIRCLE('',#14628,1.00181590545205) ;
#5236=CIRCLE('',#14629,1.1) ;
#5237=CIRCLE('',#14633,0.834979872033575) ;
#5238=CIRCLE('',#14636,1.00181590545205) ;
#5239=CIRCLE('',#14637,1.00181590545205) ;
#5240=CIRCLE('',#14639,1.1) ;
#5241=CIRCLE('',#14640,1.1) ;
#5242=CIRCLE('',#14642,1.00181590545205) ;
#5243=CIRCLE('',#14643,1.4) ;
#5244=CIRCLE('',#14645,1.00181590545205) ;
#5245=CIRCLE('',#14646,1.1) ;
#5246=CIRCLE('',#14647,1.00181590545205) ;
#5247=CIRCLE('',#14648,1.1) ;
#5248=CIRCLE('',#14652,1.4) ;
#5249=CIRCLE('',#14653,1.4) ;
#5250=CIRCLE('',#14654,1.4) ;
#5251=CIRCLE('',#14655,1.4) ;
#5252=CIRCLE('',#14657,1.4) ;
#5253=CIRCLE('',#14658,1.4) ;
#5254=CIRCLE('',#14659,1.4) ;
#5255=CIRCLE('',#14660,1.4) ;
#5256=CIRCLE('',#14662,1.4) ;
#5257=CIRCLE('',#14663,1.4) ;
#5258=CIRCLE('',#14664,1.4) ;
#5259=CIRCLE('',#14665,1.4) ;
#5260=CIRCLE('',#14667,1.4) ;
#5261=CIRCLE('',#14668,1.4) ;
#5262=CIRCLE('',#14669,1.4) ;
#5263=CIRCLE('',#14670,1.4) ;
#5264=CIRCLE('',#14672,1.4) ;
#5265=CIRCLE('',#14673,1.4) ;
#5266=CIRCLE('',#14674,1.4) ;
#5267=CIRCLE('',#14675,1.4) ;
#5268=CIRCLE('',#14677,1.4) ;
#5269=CIRCLE('',#14678,1.4) ;
#5270=CIRCLE('',#14679,1.4) ;
#5271=CIRCLE('',#14680,1.4) ;
#5272=CIRCLE('',#14682,1.4) ;
#5273=CIRCLE('',#14683,1.1) ;
#5274=CIRCLE('',#14685,1.4) ;
#5275=CIRCLE('',#14686,1.4) ;
#5276=CIRCLE('',#14687,1.4) ;
#5277=CIRCLE('',#14688,1.4) ;
#5278=CIRCLE('',#14690,1.1) ;
#5279=CIRCLE('',#14692,1.4) ;
#5280=CIRCLE('',#14694,1.4) ;
#5281=CIRCLE('',#14695,1.4) ;
#5282=CIRCLE('',#14698,1.1) ;
#5283=CIRCLE('',#14701,1.4) ;
#5284=CIRCLE('',#14703,1.4) ;
#5285=CIRCLE('',#14705,1.4) ;
#5286=CIRCLE('',#14707,1.4) ;
#5287=CIRCLE('',#14709,1.4) ;
#5288=CIRCLE('',#14713,1.4) ;
#5289=CIRCLE('',#14715,1.4) ;
#5290=CIRCLE('',#14717,1.4) ;
#5291=CIRCLE('',#14718,1.4) ;
#5292=CIRCLE('',#14720,1.4) ;
#5293=CIRCLE('',#14721,1.4) ;
#5294=CIRCLE('',#14723,1.4) ;
#5295=CIRCLE('',#14725,1.4) ;
#5296=CIRCLE('',#14729,1.4) ;
#5297=CIRCLE('',#14731,1.4) ;
#5298=CIRCLE('',#14733,1.4) ;
#5299=CIRCLE('',#14734,1.4) ;
#5300=CIRCLE('',#14736,1.4) ;
#5301=CIRCLE('',#14737,1.4) ;
#5302=CIRCLE('',#14739,1.4) ;
#5303=CIRCLE('',#14741,1.4) ;
#5304=CIRCLE('',#14745,1.4) ;
#5305=CIRCLE('',#14747,1.4) ;
#5306=CIRCLE('',#14749,1.4) ;
#5307=CIRCLE('',#14750,1.4) ;
#5308=CIRCLE('',#14752,1.4) ;
#5309=CIRCLE('',#14753,1.4) ;
#5310=CIRCLE('',#14755,1.4) ;
#5311=CIRCLE('',#14758,1.4) ;
#5312=CIRCLE('',#14761,1.4) ;
#5313=CIRCLE('',#14770,1.4) ;
#5314=CIRCLE('',#14772,1.1) ;
#5315=CIRCLE('',#14774,1.4) ;
#5316=CIRCLE('',#14777,0.834979872033575) ;
#5317=CIRCLE('',#14780,0.834979872033575) ;
#5318=CIRCLE('',#14783,0.834979872033573) ;
#5319=CIRCLE('',#14784,1.1) ;
#5320=CIRCLE('',#14786,1.1) ;
#5321=CIRCLE('',#14788,0.834979872033575) ;
#5322=CIRCLE('',#14789,1.1) ;
#5323=CIRCLE('',#14791,1.1) ;
#5324=CIRCLE('',#14793,0.834979872033573) ;
#5325=CIRCLE('',#14794,1.1) ;
#5326=CIRCLE('',#14796,1.1) ;
#5327=CIRCLE('',#14798,0.834979872033575) ;
#5328=CIRCLE('',#14799,1.1) ;
#5329=CIRCLE('',#14801,1.1) ;
#6114=VERTEX_POINT('',#21618) ;
#6115=VERTEX_POINT('',#21620) ;
#6116=VERTEX_POINT('',#21623) ;
#6117=VERTEX_POINT('',#21626) ;
#6118=VERTEX_POINT('',#21628) ;
#6119=VERTEX_POINT('',#21631) ;
#6120=VERTEX_POINT('',#21634) ;
#6121=VERTEX_POINT('',#21635) ;
#6122=VERTEX_POINT('',#21655) ;
#6123=VERTEX_POINT('',#21657) ;
#6124=VERTEX_POINT('',#21660) ;
#6125=VERTEX_POINT('',#21662) ;
#6126=VERTEX_POINT('',#21694) ;
#6127=VERTEX_POINT('',#21696) ;
#6128=VERTEX_POINT('',#21700) ;
#6129=VERTEX_POINT('',#21703) ;
#6130=VERTEX_POINT('',#21706) ;
#6131=VERTEX_POINT('',#21708) ;
#6132=VERTEX_POINT('',#21711) ;
#6133=VERTEX_POINT('',#21714) ;
#6134=VERTEX_POINT('',#21716) ;
#6135=VERTEX_POINT('',#21719) ;
#6136=VERTEX_POINT('',#21723) ;
#6137=VERTEX_POINT('',#21726) ;
#6138=VERTEX_POINT('',#21728) ;
#6139=VERTEX_POINT('',#21732) ;
#6140=VERTEX_POINT('',#21735) ;
#6141=VERTEX_POINT('',#21738) ;
#6142=VERTEX_POINT('',#21740) ;
#6143=VERTEX_POINT('',#21743) ;
#6144=VERTEX_POINT('',#21746) ;
#6145=VERTEX_POINT('',#21748) ;
#6146=VERTEX_POINT('',#21751) ;
#6147=VERTEX_POINT('',#21755) ;
#6148=VERTEX_POINT('',#21758) ;
#6149=VERTEX_POINT('',#21760) ;
#6150=VERTEX_POINT('',#21764) ;
#6151=VERTEX_POINT('',#21767) ;
#6152=VERTEX_POINT('',#21770) ;
#6153=VERTEX_POINT('',#21772) ;
#6154=VERTEX_POINT('',#21775) ;
#6155=VERTEX_POINT('',#21778) ;
#6156=VERTEX_POINT('',#21780) ;
#6157=VERTEX_POINT('',#21783) ;
#6158=VERTEX_POINT('',#21787) ;
#6159=VERTEX_POINT('',#21790) ;
#6160=VERTEX_POINT('',#21792) ;
#6161=VERTEX_POINT('',#21796) ;
#6162=VERTEX_POINT('',#21800) ;
#6163=VERTEX_POINT('',#21804) ;
#6164=VERTEX_POINT('',#21807) ;
#6165=VERTEX_POINT('',#21812) ;
#6166=VERTEX_POINT('',#21814) ;
#6167=VERTEX_POINT('',#21816) ;
#6168=VERTEX_POINT('',#21821) ;
#6169=VERTEX_POINT('',#21825) ;
#6170=VERTEX_POINT('',#21828) ;
#6171=VERTEX_POINT('',#21829) ;
#6172=VERTEX_POINT('',#21831) ;
#6173=VERTEX_POINT('',#21834) ;
#6174=VERTEX_POINT('',#21838) ;
#6175=VERTEX_POINT('',#21839) ;
#6176=VERTEX_POINT('',#21841) ;
#6177=VERTEX_POINT('',#21844) ;
#6178=VERTEX_POINT('',#21846) ;
#6179=VERTEX_POINT('',#21851) ;
#6180=VERTEX_POINT('',#21855) ;
#6181=VERTEX_POINT('',#21856) ;
#6182=VERTEX_POINT('',#21872) ;
#6183=VERTEX_POINT('',#21876) ;
#6184=VERTEX_POINT('',#21877) ;
#6185=VERTEX_POINT('',#21881) ;
#6186=VERTEX_POINT('',#21883) ;
#6187=VERTEX_POINT('',#21886) ;
#6188=VERTEX_POINT('',#21887) ;
#6189=VERTEX_POINT('',#21891) ;
#6190=VERTEX_POINT('',#21892) ;
#6191=VERTEX_POINT('',#21894) ;
#6192=VERTEX_POINT('',#21897) ;
#6193=VERTEX_POINT('',#21924) ;
#6194=VERTEX_POINT('',#21925) ;
#6195=VERTEX_POINT('',#21927) ;
#6196=VERTEX_POINT('',#21929) ;
#6197=VERTEX_POINT('',#21933) ;
#6198=VERTEX_POINT('',#21934) ;
#6199=VERTEX_POINT('',#21936) ;
#6200=VERTEX_POINT('',#21938) ;
#6201=VERTEX_POINT('',#21942) ;
#6202=VERTEX_POINT('',#21943) ;
#6203=VERTEX_POINT('',#21945) ;
#6204=VERTEX_POINT('',#21947) ;
#6205=VERTEX_POINT('',#21951) ;
#6206=VERTEX_POINT('',#21952) ;
#6207=VERTEX_POINT('',#21954) ;
#6208=VERTEX_POINT('',#21956) ;
#6209=VERTEX_POINT('',#21960) ;
#6210=VERTEX_POINT('',#21961) ;
#6211=VERTEX_POINT('',#21963) ;
#6212=VERTEX_POINT('',#21965) ;
#6213=VERTEX_POINT('',#21969) ;
#6214=VERTEX_POINT('',#21970) ;
#6215=VERTEX_POINT('',#21972) ;
#6216=VERTEX_POINT('',#21974) ;
#6217=VERTEX_POINT('',#21978) ;
#6218=VERTEX_POINT('',#21979) ;
#6219=VERTEX_POINT('',#21983) ;
#6220=VERTEX_POINT('',#21984) ;
#6221=VERTEX_POINT('',#21986) ;
#6222=VERTEX_POINT('',#21988) ;
#6223=VERTEX_POINT('',#21992) ;
#6224=VERTEX_POINT('',#21994) ;
#6225=VERTEX_POINT('',#22027) ;
#6226=VERTEX_POINT('',#22029) ;
#6227=VERTEX_POINT('',#22031) ;
#6228=VERTEX_POINT('',#22033) ;
#6229=VERTEX_POINT('',#22035) ;
#6230=VERTEX_POINT('',#22039) ;
#6231=VERTEX_POINT('',#22042) ;
#6232=VERTEX_POINT('',#22044) ;
#6233=VERTEX_POINT('',#22046) ;
#6234=VERTEX_POINT('',#22051) ;
#6235=VERTEX_POINT('',#22052) ;
#6236=VERTEX_POINT('',#22067) ;
#6237=VERTEX_POINT('',#22086) ;
#6238=VERTEX_POINT('',#22095) ;
#6239=VERTEX_POINT('',#22097) ;
#6240=VERTEX_POINT('',#22099) ;
#6241=VERTEX_POINT('',#22103) ;
#6242=VERTEX_POINT('',#22105) ;
#6243=VERTEX_POINT('',#22107) ;
#6244=VERTEX_POINT('',#22109) ;
#6245=VERTEX_POINT('',#22114) ;
#6246=VERTEX_POINT('',#22123) ;
#6247=VERTEX_POINT('',#22125) ;
#6248=VERTEX_POINT('',#22127) ;
#6249=VERTEX_POINT('',#22131) ;
#6250=VERTEX_POINT('',#22133) ;
#6251=VERTEX_POINT('',#22135) ;
#6252=VERTEX_POINT('',#22137) ;
#6253=VERTEX_POINT('',#22142) ;
#6254=VERTEX_POINT('',#22151) ;
#6255=VERTEX_POINT('',#22153) ;
#6256=VERTEX_POINT('',#22155) ;
#6257=VERTEX_POINT('',#22159) ;
#6258=VERTEX_POINT('',#22161) ;
#6259=VERTEX_POINT('',#22163) ;
#6260=VERTEX_POINT('',#22165) ;
#6261=VERTEX_POINT('',#22170) ;
#6262=VERTEX_POINT('',#22173) ;
#6263=VERTEX_POINT('',#22179) ;
#6264=VERTEX_POINT('',#22190) ;
#6265=VERTEX_POINT('',#22196) ;
#6266=VERTEX_POINT('',#22200) ;
#6267=VERTEX_POINT('',#22204) ;
#6268=VERTEX_POINT('',#22208) ;
#6269=VERTEX_POINT('',#22210) ;
#6270=VERTEX_POINT('',#22213) ;
#6271=VERTEX_POINT('',#22216) ;
#6272=VERTEX_POINT('',#22218) ;
#6273=VERTEX_POINT('',#22221) ;
#6274=VERTEX_POINT('',#22224) ;
#6275=VERTEX_POINT('',#22226) ;
#6276=VERTEX_POINT('',#22229) ;
#6277=VERTEX_POINT('',#22232) ;
#6278=VERTEX_POINT('',#22234) ;
#6279=VERTEX_POINT('',#22237) ;
#7592=EDGE_CURVE('',#6114,#6114,#5160,.T.) ;
#7593=EDGE_CURVE('',#6114,#6115,#5161,.T.) ;
#7594=EDGE_CURVE('',#6116,#6114,#5162,.T.) ;
#7595=EDGE_CURVE('',#6117,#6117,#5163,.T.) ;
#7596=EDGE_CURVE('',#6118,#6117,#5164,.T.) ;
#7597=EDGE_CURVE('',#6117,#6119,#5165,.T.) ;
#7598=EDGE_CURVE('',#6120,#6121,#5166,.T.) ;
#7599=EDGE_CURVE('',#6121,#6120,#956,.T.) ;
#7600=EDGE_CURVE('',#6120,#6121,#5167,.T.) ;
#7601=EDGE_CURVE('',#6122,#6122,#5168,.T.) ;
#7602=EDGE_CURVE('',#6123,#6122,#5169,.T.) ;
#7603=EDGE_CURVE('',#6122,#6124,#5170,.T.) ;
#7604=EDGE_CURVE('',#6125,#6124,#957,.T.) ;
#7605=EDGE_CURVE('',#6124,#6125,#5171,.T.) ;
#7606=EDGE_CURVE('',#6125,#6124,#5172,.T.) ;
#7607=EDGE_CURVE('',#6126,#6126,#5173,.T.) ;
#7608=EDGE_CURVE('',#6126,#6127,#5174,.T.) ;
#7609=EDGE_CURVE('',#6127,#6127,#5175,.T.) ;
#7610=EDGE_CURVE('',#6127,#6128,#5176,.T.) ;
#7611=EDGE_CURVE('',#6129,#6126,#5177,.T.) ;
#7612=EDGE_CURVE('',#6130,#6130,#5178,.T.) ;
#7613=EDGE_CURVE('',#6131,#6130,#5179,.T.) ;
#7614=EDGE_CURVE('',#6130,#6132,#5180,.T.) ;
#7615=EDGE_CURVE('',#6133,#6133,#5181,.T.) ;
#7616=EDGE_CURVE('',#6134,#6133,#5182,.T.) ;
#7617=EDGE_CURVE('',#6133,#6135,#5183,.T.) ;
#7618=EDGE_CURVE('',#6135,#6135,#5184,.T.) ;
#7619=EDGE_CURVE('',#6135,#6136,#5185,.T.) ;
#7620=EDGE_CURVE('',#6137,#6137,#5186,.T.) ;
#7621=EDGE_CURVE('',#6137,#6138,#5187,.T.) ;
#7622=EDGE_CURVE('',#6138,#6138,#5188,.T.) ;
#7623=EDGE_CURVE('',#6138,#6139,#5189,.T.) ;
#7624=EDGE_CURVE('',#6140,#6137,#5190,.T.) ;
#7625=EDGE_CURVE('',#6141,#6141,#5191,.T.) ;
#7626=EDGE_CURVE('',#6142,#6141,#5192,.T.) ;
#7627=EDGE_CURVE('',#6141,#6143,#5193,.T.) ;
#7628=EDGE_CURVE('',#6144,#6144,#5194,.T.) ;
#7629=EDGE_CURVE('',#6145,#6144,#5195,.T.) ;
#7630=EDGE_CURVE('',#6144,#6146,#5196,.T.) ;
#7631=EDGE_CURVE('',#6146,#6146,#5197,.T.) ;
#7632=EDGE_CURVE('',#6146,#6147,#5198,.T.) ;
#7633=EDGE_CURVE('',#6148,#6148,#5199,.T.) ;
#7634=EDGE_CURVE('',#6148,#6149,#5200,.T.) ;
#7635=EDGE_CURVE('',#6149,#6149,#5201,.T.) ;
#7636=EDGE_CURVE('',#6149,#6150,#5202,.T.) ;
#7637=EDGE_CURVE('',#6151,#6148,#5203,.T.) ;
#7638=EDGE_CURVE('',#6152,#6152,#5204,.T.) ;
#7639=EDGE_CURVE('',#6153,#6152,#5205,.T.) ;
#7640=EDGE_CURVE('',#6152,#6154,#5206,.T.) ;
#7641=EDGE_CURVE('',#6155,#6155,#5207,.T.) ;
#7642=EDGE_CURVE('',#6156,#6155,#5208,.T.) ;
#7643=EDGE_CURVE('',#6155,#6157,#5209,.T.) ;
#7644=EDGE_CURVE('',#6157,#6157,#5210,.T.) ;
#7645=EDGE_CURVE('',#6157,#6158,#5211,.T.) ;
#7646=EDGE_CURVE('',#6159,#6159,#5212,.T.) ;
#7647=EDGE_CURVE('',#6159,#6160,#5213,.T.) ;
#7648=EDGE_CURVE('',#6160,#6160,#5214,.T.) ;
#7649=EDGE_CURVE('',#6160,#6161,#5215,.T.) ;
#7650=EDGE_CURVE('',#6162,#6162,#5216,.T.) ;
#7651=EDGE_CURVE('',#6163,#6163,#5217,.T.) ;
#7652=EDGE_CURVE('',#6163,#6164,#5218,.T.) ;
#7653=EDGE_CURVE('',#6164,#6164,#5219,.T.) ;
#7654=EDGE_CURVE('',#6165,#6165,#5220,.T.) ;
#7655=EDGE_CURVE('',#6166,#6165,#5221,.T.) ;
#7656=EDGE_CURVE('',#6167,#6167,#5222,.T.) ;
#7657=EDGE_CURVE('',#6168,#6168,#5223,.T.) ;
#7658=EDGE_CURVE('',#6169,#6169,#5224,.T.) ;
#7659=EDGE_CURVE('',#6170,#6171,#5225,.T.) ;
#7660=EDGE_CURVE('',#6172,#6170,#5226,.T.) ;
#7661=EDGE_CURVE('',#6171,#6170,#5227,.T.) ;
#7662=EDGE_CURVE('',#6171,#6173,#5228,.T.) ;
#7663=EDGE_CURVE('',#6174,#6175,#5229,.T.) ;
#7664=EDGE_CURVE('',#6176,#6174,#5230,.T.) ;
#7665=EDGE_CURVE('',#6175,#6174,#5231,.T.) ;
#7666=EDGE_CURVE('',#6175,#6177,#5232,.T.) ;
#7667=EDGE_CURVE('',#6178,#6178,#5233,.T.) ;
#7668=EDGE_CURVE('',#6179,#6179,#5234,.T.) ;
#7669=EDGE_CURVE('',#6180,#6181,#5235,.T.) ;
#7670=EDGE_CURVE('',#6181,#6180,#5236,.T.) ;
#7671=EDGE_CURVE('',#6180,#6181,#958,.T.) ;
#7672=EDGE_CURVE('',#6182,#6182,#5237,.T.) ;
#7673=EDGE_CURVE('',#6183,#6184,#5238,.T.) ;
#7674=EDGE_CURVE('',#6184,#6183,#5239,.T.) ;
#7675=EDGE_CURVE('',#6185,#6183,#5240,.T.) ;
#7676=EDGE_CURVE('',#6184,#6186,#5241,.T.) ;
#7677=EDGE_CURVE('',#6187,#6188,#5242,.T.) ;
#7678=EDGE_CURVE('',#6187,#6188,#5243,.T.) ;
#7679=EDGE_CURVE('',#6189,#6190,#5244,.T.) ;
#7680=EDGE_CURVE('',#6191,#6189,#5245,.T.) ;
#7681=EDGE_CURVE('',#6190,#6189,#5246,.T.) ;
#7682=EDGE_CURVE('',#6190,#6192,#5247,.T.) ;
#7683=EDGE_CURVE('',#6187,#6188,#959,.T.) ;
#7684=EDGE_CURVE('',#6193,#6194,#5248,.T.) ;
#7685=EDGE_CURVE('',#6194,#6195,#5249,.T.) ;
#7686=EDGE_CURVE('',#6195,#6196,#5250,.T.) ;
#7687=EDGE_CURVE('',#6196,#6193,#5251,.T.) ;
#7688=EDGE_CURVE('',#6197,#6198,#5252,.T.) ;
#7689=EDGE_CURVE('',#6198,#6199,#5253,.T.) ;
#7690=EDGE_CURVE('',#6199,#6200,#5254,.T.) ;
#7691=EDGE_CURVE('',#6200,#6197,#5255,.T.) ;
#7692=EDGE_CURVE('',#6201,#6202,#5256,.T.) ;
#7693=EDGE_CURVE('',#6202,#6203,#5257,.T.) ;
#7694=EDGE_CURVE('',#6203,#6204,#5258,.T.) ;
#7695=EDGE_CURVE('',#6204,#6201,#5259,.T.) ;
#7696=EDGE_CURVE('',#6205,#6206,#5260,.T.) ;
#7697=EDGE_CURVE('',#6206,#6207,#5261,.T.) ;
#7698=EDGE_CURVE('',#6207,#6208,#5262,.T.) ;
#7699=EDGE_CURVE('',#6208,#6205,#5263,.T.) ;
#7700=EDGE_CURVE('',#6209,#6210,#5264,.T.) ;
#7701=EDGE_CURVE('',#6210,#6211,#5265,.T.) ;
#7702=EDGE_CURVE('',#6211,#6212,#5266,.T.) ;
#7703=EDGE_CURVE('',#6212,#6209,#5267,.T.) ;
#7704=EDGE_CURVE('',#6213,#6214,#5268,.T.) ;
#7705=EDGE_CURVE('',#6214,#6215,#5269,.T.) ;
#7706=EDGE_CURVE('',#6215,#6216,#5270,.T.) ;
#7707=EDGE_CURVE('',#6216,#6213,#5271,.T.) ;
#7708=EDGE_CURVE('',#6217,#6218,#5272,.T.) ;
#7709=EDGE_CURVE('',#6217,#6218,#5273,.T.) ;
#7710=EDGE_CURVE('',#6219,#6220,#5274,.T.) ;
#7711=EDGE_CURVE('',#6221,#6220,#5275,.T.) ;
#7712=EDGE_CURVE('',#6220,#6222,#5276,.T.) ;
#7713=EDGE_CURVE('',#6222,#6219,#5277,.T.) ;
#7714=EDGE_CURVE('',#6223,#6223,#5278,.T.) ;
#7715=EDGE_CURVE('',#6223,#6224,#1388,.T.) ;
#7716=EDGE_CURVE('',#6224,#6217,#960,.T.) ;
#7717=EDGE_CURVE('',#6218,#6224,#961,.T.) ;
#7718=EDGE_CURVE('',#6225,#6225,#5279,.T.) ;
#7719=EDGE_CURVE('',#6225,#6226,#1389,.T.) ;
#7720=EDGE_CURVE('',#6227,#6226,#335,.T.) ;
#7721=EDGE_CURVE('',#6228,#6227,#5280,.T.) ;
#7722=EDGE_CURVE('',#6229,#6228,#5281,.T.) ;
#7723=EDGE_CURVE('',#6226,#6229,#336,.T.) ;
#7724=EDGE_CURVE('',#6230,#6230,#5282,.T.) ;
#7725=EDGE_CURVE('',#6229,#6231,#1390,.T.) ;
#7726=EDGE_CURVE('',#6232,#6231,#337,.T.) ;
#7727=EDGE_CURVE('',#6233,#6232,#5283,.T.) ;
#7728=EDGE_CURVE('',#6231,#6233,#338,.T.) ;
#7729=EDGE_CURVE('',#6227,#6229,#5284,.T.) ;
#7730=EDGE_CURVE('',#6234,#6235,#962,.T.) ;
#7731=EDGE_CURVE('',#6235,#6236,#963,.T.) ;
#7732=EDGE_CURVE('',#6234,#6236,#5285,.T.) ;
#7733=EDGE_CURVE('',#6237,#6233,#5286,.T.) ;
#7734=EDGE_CURVE('',#6237,#6194,#1391,.T.) ;
#7735=EDGE_CURVE('',#6195,#6193,#339,.T.) ;
#7736=EDGE_CURVE('',#6232,#6237,#5287,.T.) ;
#7737=EDGE_CURVE('',#6196,#6198,#1392,.T.) ;
#7738=EDGE_CURVE('',#6199,#6197,#340,.T.) ;
#7739=EDGE_CURVE('',#6200,#6238,#1393,.T.) ;
#7740=EDGE_CURVE('',#6239,#6238,#5288,.T.) ;
#7741=EDGE_CURVE('',#6240,#6239,#341,.T.) ;
#7742=EDGE_CURVE('',#6238,#6240,#5289,.T.) ;
#7743=EDGE_CURVE('',#6241,#6239,#5290,.T.) ;
#7744=EDGE_CURVE('',#6241,#6242,#1394,.T.) ;
#7745=EDGE_CURVE('',#6243,#6242,#5291,.T.) ;
#7746=EDGE_CURVE('',#6244,#6243,#342,.T.) ;
#7747=EDGE_CURVE('',#6242,#6244,#5292,.T.) ;
#7748=EDGE_CURVE('',#6240,#6241,#5293,.T.) ;
#7749=EDGE_CURVE('',#6245,#6243,#5294,.T.) ;
#7750=EDGE_CURVE('',#6245,#6202,#1395,.T.) ;
#7751=EDGE_CURVE('',#6203,#6201,#343,.T.) ;
#7752=EDGE_CURVE('',#6244,#6245,#5295,.T.) ;
#7753=EDGE_CURVE('',#6204,#6206,#1396,.T.) ;
#7754=EDGE_CURVE('',#6207,#6205,#344,.T.) ;
#7755=EDGE_CURVE('',#6208,#6246,#1397,.T.) ;
#7756=EDGE_CURVE('',#6247,#6246,#5296,.T.) ;
#7757=EDGE_CURVE('',#6248,#6247,#345,.T.) ;
#7758=EDGE_CURVE('',#6246,#6248,#5297,.T.) ;
#7759=EDGE_CURVE('',#6249,#6247,#5298,.T.) ;
#7760=EDGE_CURVE('',#6249,#6250,#1398,.T.) ;
#7761=EDGE_CURVE('',#6251,#6250,#5299,.T.) ;
#7762=EDGE_CURVE('',#6252,#6251,#346,.T.) ;
#7763=EDGE_CURVE('',#6250,#6252,#5300,.T.) ;
#7764=EDGE_CURVE('',#6248,#6249,#5301,.T.) ;
#7765=EDGE_CURVE('',#6253,#6251,#5302,.T.) ;
#7766=EDGE_CURVE('',#6253,#6210,#1399,.T.) ;
#7767=EDGE_CURVE('',#6211,#6209,#347,.T.) ;
#7768=EDGE_CURVE('',#6252,#6253,#5303,.T.) ;
#7769=EDGE_CURVE('',#6212,#6214,#1400,.T.) ;
#7770=EDGE_CURVE('',#6215,#6213,#348,.T.) ;
#7771=EDGE_CURVE('',#6216,#6254,#1401,.T.) ;
#7772=EDGE_CURVE('',#6255,#6254,#5304,.T.) ;
#7773=EDGE_CURVE('',#6256,#6255,#349,.T.) ;
#7774=EDGE_CURVE('',#6254,#6256,#5305,.T.) ;
#7775=EDGE_CURVE('',#6257,#6255,#5306,.T.) ;
#7776=EDGE_CURVE('',#6257,#6258,#1402,.T.) ;
#7777=EDGE_CURVE('',#6259,#6258,#5307,.T.) ;
#7778=EDGE_CURVE('',#6260,#6259,#350,.T.) ;
#7779=EDGE_CURVE('',#6258,#6260,#5308,.T.) ;
#7780=EDGE_CURVE('',#6256,#6257,#5309,.T.) ;
#7781=EDGE_CURVE('',#6261,#6259,#5310,.T.) ;
#7782=EDGE_CURVE('',#6261,#6222,#1403,.T.) ;
#7783=EDGE_CURVE('',#6262,#6219,#351,.T.) ;
#7784=EDGE_CURVE('',#6222,#6262,#352,.T.) ;
#7785=EDGE_CURVE('',#6260,#6261,#5311,.T.) ;
#7786=EDGE_CURVE('',#6262,#6263,#1404,.T.) ;
#7787=EDGE_CURVE('',#6263,#6263,#5312,.T.) ;
#7788=EDGE_CURVE('',#6237,#6264,#5313,.T.) ;
#7789=EDGE_CURVE('',#6234,#6236,#5314,.T.) ;
#7790=EDGE_CURVE('',#6235,#6230,#1405,.T.) ;
#7791=EDGE_CURVE('',#6265,#6228,#5315,.T.) ;
#7792=EDGE_CURVE('',#6266,#6266,#5316,.T.) ;
#7793=EDGE_CURVE('',#6267,#6267,#5317,.T.) ;
#7794=EDGE_CURVE('',#6268,#6268,#5318,.T.) ;
#7795=EDGE_CURVE('',#6268,#6269,#5319,.T.) ;
#7796=EDGE_CURVE('',#6270,#6268,#5320,.T.) ;
#7797=EDGE_CURVE('',#6271,#6271,#5321,.T.) ;
#7798=EDGE_CURVE('',#6271,#6272,#5322,.T.) ;
#7799=EDGE_CURVE('',#6273,#6271,#5323,.T.) ;
#7800=EDGE_CURVE('',#6274,#6274,#5324,.T.) ;
#7801=EDGE_CURVE('',#6274,#6275,#5325,.T.) ;
#7802=EDGE_CURVE('',#6276,#6274,#5326,.T.) ;
#7803=EDGE_CURVE('',#6277,#6277,#5327,.T.) ;
#7804=EDGE_CURVE('',#6277,#6278,#5328,.T.) ;
#7805=EDGE_CURVE('',#6279,#6277,#5329,.T.) ;
#10205=ORIENTED_EDGE('',*,*,#7592,.T.) ;
#10206=ORIENTED_EDGE('',*,*,#7593,.T.) ;
#10207=ORIENTED_EDGE('',*,*,#7593,.F.) ;
#10208=ORIENTED_EDGE('',*,*,#7592,.F.) ;
#10209=ORIENTED_EDGE('',*,*,#7594,.F.) ;
#10210=ORIENTED_EDGE('',*,*,#7594,.T.) ;
#10211=ORIENTED_EDGE('',*,*,#7595,.T.) ;
#10212=ORIENTED_EDGE('',*,*,#7596,.F.) ;
#10213=ORIENTED_EDGE('',*,*,#7596,.T.) ;
#10214=ORIENTED_EDGE('',*,*,#7595,.F.) ;
#10215=ORIENTED_EDGE('',*,*,#7597,.T.) ;
#10216=ORIENTED_EDGE('',*,*,#7597,.F.) ;
#10217=ORIENTED_EDGE('',*,*,#7598,.F.) ;
#10218=ORIENTED_EDGE('',*,*,#7599,.F.) ;
#10219=ORIENTED_EDGE('',*,*,#7599,.T.) ;
#10220=ORIENTED_EDGE('',*,*,#7600,.T.) ;
#10221=ORIENTED_EDGE('',*,*,#7598,.T.) ;
#10222=ORIENTED_EDGE('',*,*,#7600,.F.) ;
#10223=ORIENTED_EDGE('',*,*,#7601,.F.) ;
#10224=ORIENTED_EDGE('',*,*,#7602,.F.) ;
#10225=ORIENTED_EDGE('',*,*,#7602,.T.) ;
#10226=ORIENTED_EDGE('',*,*,#7601,.T.) ;
#10227=ORIENTED_EDGE('',*,*,#7603,.T.) ;
#10228=ORIENTED_EDGE('',*,*,#7604,.F.) ;
#10229=ORIENTED_EDGE('',*,*,#7605,.F.) ;
#10230=ORIENTED_EDGE('',*,*,#7603,.F.) ;
#10231=ORIENTED_EDGE('',*,*,#7605,.T.) ;
#10232=ORIENTED_EDGE('',*,*,#7606,.T.) ;
#10233=ORIENTED_EDGE('',*,*,#7604,.T.) ;
#10234=ORIENTED_EDGE('',*,*,#7606,.F.) ;
#10235=ORIENTED_EDGE('',*,*,#7607,.T.) ;
#10236=ORIENTED_EDGE('',*,*,#7608,.T.) ;
#10237=ORIENTED_EDGE('',*,*,#7609,.F.) ;
#10238=ORIENTED_EDGE('',*,*,#7608,.F.) ;
#10239=ORIENTED_EDGE('',*,*,#7609,.T.) ;
#10240=ORIENTED_EDGE('',*,*,#7610,.T.) ;
#10241=ORIENTED_EDGE('',*,*,#7610,.F.) ;
#10242=ORIENTED_EDGE('',*,*,#7607,.F.) ;
#10243=ORIENTED_EDGE('',*,*,#7611,.F.) ;
#10244=ORIENTED_EDGE('',*,*,#7611,.T.) ;
#10245=ORIENTED_EDGE('',*,*,#7612,.T.) ;
#10246=ORIENTED_EDGE('',*,*,#7613,.F.) ;
#10247=ORIENTED_EDGE('',*,*,#7613,.T.) ;
#10248=ORIENTED_EDGE('',*,*,#7612,.F.) ;
#10249=ORIENTED_EDGE('',*,*,#7614,.T.) ;
#10250=ORIENTED_EDGE('',*,*,#7614,.F.) ;
#10251=ORIENTED_EDGE('',*,*,#7615,.F.) ;
#10252=ORIENTED_EDGE('',*,*,#7616,.F.) ;
#10253=ORIENTED_EDGE('',*,*,#7616,.T.) ;
#10254=ORIENTED_EDGE('',*,*,#7615,.T.) ;
#10255=ORIENTED_EDGE('',*,*,#7617,.T.) ;
#10256=ORIENTED_EDGE('',*,*,#7618,.F.) ;
#10257=ORIENTED_EDGE('',*,*,#7617,.F.) ;
#10258=ORIENTED_EDGE('',*,*,#7618,.T.) ;
#10259=ORIENTED_EDGE('',*,*,#7619,.T.) ;
#10260=ORIENTED_EDGE('',*,*,#7619,.F.) ;
#10261=ORIENTED_EDGE('',*,*,#7620,.T.) ;
#10262=ORIENTED_EDGE('',*,*,#7621,.T.) ;
#10263=ORIENTED_EDGE('',*,*,#7622,.F.) ;
#10264=ORIENTED_EDGE('',*,*,#7621,.F.) ;
#10265=ORIENTED_EDGE('',*,*,#7622,.T.) ;
#10266=ORIENTED_EDGE('',*,*,#7623,.T.) ;
#10267=ORIENTED_EDGE('',*,*,#7623,.F.) ;
#10268=ORIENTED_EDGE('',*,*,#7620,.F.) ;
#10269=ORIENTED_EDGE('',*,*,#7624,.F.) ;
#10270=ORIENTED_EDGE('',*,*,#7624,.T.) ;
#10271=ORIENTED_EDGE('',*,*,#7625,.T.) ;
#10272=ORIENTED_EDGE('',*,*,#7626,.F.) ;
#10273=ORIENTED_EDGE('',*,*,#7626,.T.) ;
#10274=ORIENTED_EDGE('',*,*,#7625,.F.) ;
#10275=ORIENTED_EDGE('',*,*,#7627,.T.) ;
#10276=ORIENTED_EDGE('',*,*,#7627,.F.) ;
#10277=ORIENTED_EDGE('',*,*,#7628,.F.) ;
#10278=ORIENTED_EDGE('',*,*,#7629,.F.) ;
#10279=ORIENTED_EDGE('',*,*,#7629,.T.) ;
#10280=ORIENTED_EDGE('',*,*,#7628,.T.) ;
#10281=ORIENTED_EDGE('',*,*,#7630,.T.) ;
#10282=ORIENTED_EDGE('',*,*,#7631,.F.) ;
#10283=ORIENTED_EDGE('',*,*,#7630,.F.) ;
#10284=ORIENTED_EDGE('',*,*,#7631,.T.) ;
#10285=ORIENTED_EDGE('',*,*,#7632,.T.) ;
#10286=ORIENTED_EDGE('',*,*,#7632,.F.) ;
#10287=ORIENTED_EDGE('',*,*,#7633,.T.) ;
#10288=ORIENTED_EDGE('',*,*,#7634,.T.) ;
#10289=ORIENTED_EDGE('',*,*,#7635,.F.) ;
#10290=ORIENTED_EDGE('',*,*,#7634,.F.) ;
#10291=ORIENTED_EDGE('',*,*,#7635,.T.) ;
#10292=ORIENTED_EDGE('',*,*,#7636,.T.) ;
#10293=ORIENTED_EDGE('',*,*,#7636,.F.) ;
#10294=ORIENTED_EDGE('',*,*,#7633,.F.) ;
#10295=ORIENTED_EDGE('',*,*,#7637,.F.) ;
#10296=ORIENTED_EDGE('',*,*,#7637,.T.) ;
#10297=ORIENTED_EDGE('',*,*,#7638,.T.) ;
#10298=ORIENTED_EDGE('',*,*,#7639,.F.) ;
#10299=ORIENTED_EDGE('',*,*,#7639,.T.) ;
#10300=ORIENTED_EDGE('',*,*,#7638,.F.) ;
#10301=ORIENTED_EDGE('',*,*,#7640,.T.) ;
#10302=ORIENTED_EDGE('',*,*,#7640,.F.) ;
#10303=ORIENTED_EDGE('',*,*,#7641,.F.) ;
#10304=ORIENTED_EDGE('',*,*,#7642,.F.) ;
#10305=ORIENTED_EDGE('',*,*,#7642,.T.) ;
#10306=ORIENTED_EDGE('',*,*,#7641,.T.) ;
#10307=ORIENTED_EDGE('',*,*,#7643,.T.) ;
#10308=ORIENTED_EDGE('',*,*,#7644,.F.) ;
#10309=ORIENTED_EDGE('',*,*,#7643,.F.) ;
#10310=ORIENTED_EDGE('',*,*,#7644,.T.) ;
#10311=ORIENTED_EDGE('',*,*,#7645,.T.) ;
#10312=ORIENTED_EDGE('',*,*,#7645,.F.) ;
#10313=ORIENTED_EDGE('',*,*,#7646,.T.) ;
#10314=ORIENTED_EDGE('',*,*,#7647,.T.) ;
#10315=ORIENTED_EDGE('',*,*,#7648,.F.) ;
#10316=ORIENTED_EDGE('',*,*,#7647,.F.) ;
#10317=ORIENTED_EDGE('',*,*,#7648,.T.) ;
#10318=ORIENTED_EDGE('',*,*,#7649,.T.) ;
#10319=ORIENTED_EDGE('',*,*,#7649,.F.) ;
#10320=ORIENTED_EDGE('',*,*,#7646,.F.) ;
#10321=ORIENTED_EDGE('',*,*,#7650,.T.) ;
#10322=ORIENTED_EDGE('',*,*,#7650,.F.) ;
#10323=ORIENTED_EDGE('',*,*,#7651,.F.) ;
#10324=ORIENTED_EDGE('',*,*,#7651,.T.) ;
#10325=ORIENTED_EDGE('',*,*,#7652,.T.) ;
#10326=ORIENTED_EDGE('',*,*,#7653,.F.) ;
#10327=ORIENTED_EDGE('',*,*,#7652,.F.) ;
#10328=ORIENTED_EDGE('',*,*,#7653,.T.) ;
#10329=ORIENTED_EDGE('',*,*,#7654,.F.) ;
#10330=ORIENTED_EDGE('',*,*,#7655,.F.) ;
#10331=ORIENTED_EDGE('',*,*,#7655,.T.) ;
#10332=ORIENTED_EDGE('',*,*,#7656,.T.) ;
#10333=ORIENTED_EDGE('',*,*,#7654,.T.) ;
#10334=ORIENTED_EDGE('',*,*,#7656,.F.) ;
#10335=ORIENTED_EDGE('',*,*,#7657,.T.) ;
#10336=ORIENTED_EDGE('',*,*,#7657,.F.) ;
#10337=ORIENTED_EDGE('',*,*,#7658,.F.) ;
#10338=ORIENTED_EDGE('',*,*,#7659,.F.) ;
#10339=ORIENTED_EDGE('',*,*,#7660,.F.) ;
#10340=ORIENTED_EDGE('',*,*,#7660,.T.) ;
#10341=ORIENTED_EDGE('',*,*,#7661,.F.) ;
#10342=ORIENTED_EDGE('',*,*,#7662,.T.) ;
#10343=ORIENTED_EDGE('',*,*,#7662,.F.) ;
#10344=ORIENTED_EDGE('',*,*,#7658,.T.) ;
#10345=ORIENTED_EDGE('',*,*,#7659,.T.) ;
#10346=ORIENTED_EDGE('',*,*,#7661,.T.) ;
#10347=ORIENTED_EDGE('',*,*,#7663,.F.) ;
#10348=ORIENTED_EDGE('',*,*,#7664,.F.) ;
#10349=ORIENTED_EDGE('',*,*,#7664,.T.) ;
#10350=ORIENTED_EDGE('',*,*,#7665,.F.) ;
#10351=ORIENTED_EDGE('',*,*,#7666,.T.) ;
#10352=ORIENTED_EDGE('',*,*,#7666,.F.) ;
#10353=ORIENTED_EDGE('',*,*,#7667,.T.) ;
#10354=ORIENTED_EDGE('',*,*,#7663,.T.) ;
#10355=ORIENTED_EDGE('',*,*,#7665,.T.) ;
#10356=ORIENTED_EDGE('',*,*,#7667,.F.) ;
#10357=ORIENTED_EDGE('',*,*,#7668,.T.) ;
#10358=ORIENTED_EDGE('',*,*,#7668,.F.) ;
#10359=ORIENTED_EDGE('',*,*,#7669,.F.) ;
#10360=ORIENTED_EDGE('',*,*,#7670,.F.) ;
#10361=ORIENTED_EDGE('',*,*,#7670,.T.) ;
#10362=ORIENTED_EDGE('',*,*,#7671,.T.) ;
#10363=ORIENTED_EDGE('',*,*,#7669,.T.) ;
#10364=ORIENTED_EDGE('',*,*,#7671,.F.) ;
#10365=ORIENTED_EDGE('',*,*,#7672,.F.) ;
#10366=ORIENTED_EDGE('',*,*,#7672,.T.) ;
#10367=ORIENTED_EDGE('',*,*,#7673,.T.) ;
#10368=ORIENTED_EDGE('',*,*,#7674,.T.) ;
#10369=ORIENTED_EDGE('',*,*,#7673,.F.) ;
#10370=ORIENTED_EDGE('',*,*,#7675,.F.) ;
#10371=ORIENTED_EDGE('',*,*,#7675,.T.) ;
#10372=ORIENTED_EDGE('',*,*,#7674,.F.) ;
#10373=ORIENTED_EDGE('',*,*,#7676,.T.) ;
#10374=ORIENTED_EDGE('',*,*,#7676,.F.) ;
#10375=ORIENTED_EDGE('',*,*,#7677,.F.) ;
#10376=ORIENTED_EDGE('',*,*,#7678,.T.) ;
#10377=ORIENTED_EDGE('',*,*,#7679,.F.) ;
#10378=ORIENTED_EDGE('',*,*,#7680,.F.) ;
#10379=ORIENTED_EDGE('',*,*,#7680,.T.) ;
#10380=ORIENTED_EDGE('',*,*,#7681,.F.) ;
#10381=ORIENTED_EDGE('',*,*,#7682,.T.) ;
#10382=ORIENTED_EDGE('',*,*,#7682,.F.) ;
#10383=ORIENTED_EDGE('',*,*,#7677,.T.) ;
#10384=ORIENTED_EDGE('',*,*,#7683,.F.) ;
#10385=ORIENTED_EDGE('',*,*,#7683,.T.) ;
#10386=ORIENTED_EDGE('',*,*,#7678,.F.) ;
#10387=ORIENTED_EDGE('',*,*,#7679,.T.) ;
#10388=ORIENTED_EDGE('',*,*,#7681,.T.) ;
#10389=ORIENTED_EDGE('',*,*,#7684,.T.) ;
#10390=ORIENTED_EDGE('',*,*,#7685,.T.) ;
#10391=ORIENTED_EDGE('',*,*,#7686,.T.) ;
#10392=ORIENTED_EDGE('',*,*,#7687,.T.) ;
#10393=ORIENTED_EDGE('',*,*,#7688,.T.) ;
#10394=ORIENTED_EDGE('',*,*,#7689,.T.) ;
#10395=ORIENTED_EDGE('',*,*,#7690,.T.) ;
#10396=ORIENTED_EDGE('',*,*,#7691,.T.) ;
#10397=ORIENTED_EDGE('',*,*,#7692,.T.) ;
#10398=ORIENTED_EDGE('',*,*,#7693,.T.) ;
#10399=ORIENTED_EDGE('',*,*,#7694,.T.) ;
#10400=ORIENTED_EDGE('',*,*,#7695,.T.) ;
#10401=ORIENTED_EDGE('',*,*,#7696,.T.) ;
#10402=ORIENTED_EDGE('',*,*,#7697,.T.) ;
#10403=ORIENTED_EDGE('',*,*,#7698,.T.) ;
#10404=ORIENTED_EDGE('',*,*,#7699,.T.) ;
#10405=ORIENTED_EDGE('',*,*,#7700,.T.) ;
#10406=ORIENTED_EDGE('',*,*,#7701,.T.) ;
#10407=ORIENTED_EDGE('',*,*,#7702,.T.) ;
#10408=ORIENTED_EDGE('',*,*,#7703,.T.) ;
#10409=ORIENTED_EDGE('',*,*,#7704,.T.) ;
#10410=ORIENTED_EDGE('',*,*,#7705,.T.) ;
#10411=ORIENTED_EDGE('',*,*,#7706,.T.) ;
#10412=ORIENTED_EDGE('',*,*,#7707,.T.) ;
#10413=ORIENTED_EDGE('',*,*,#7708,.T.) ;
#10414=ORIENTED_EDGE('',*,*,#7709,.F.) ;
#10415=ORIENTED_EDGE('',*,*,#7710,.T.) ;
#10416=ORIENTED_EDGE('',*,*,#7711,.F.) ;
#10417=ORIENTED_EDGE('',*,*,#7711,.T.) ;
#10418=ORIENTED_EDGE('',*,*,#7712,.T.) ;
#10419=ORIENTED_EDGE('',*,*,#7713,.T.) ;
#10420=ORIENTED_EDGE('',*,*,#7714,.F.) ;
#10421=ORIENTED_EDGE('',*,*,#7715,.T.) ;
#10422=ORIENTED_EDGE('',*,*,#7716,.T.) ;
#10423=ORIENTED_EDGE('',*,*,#7709,.T.) ;
#10424=ORIENTED_EDGE('',*,*,#7717,.T.) ;
#10425=ORIENTED_EDGE('',*,*,#7715,.F.) ;
#10426=ORIENTED_EDGE('',*,*,#7718,.F.) ;
#10427=ORIENTED_EDGE('',*,*,#7719,.T.) ;
#10428=ORIENTED_EDGE('',*,*,#7720,.F.) ;
#10429=ORIENTED_EDGE('',*,*,#7721,.F.) ;
#10430=ORIENTED_EDGE('',*,*,#7722,.F.) ;
#10431=ORIENTED_EDGE('',*,*,#7723,.F.) ;
#10432=ORIENTED_EDGE('',*,*,#7719,.F.) ;
#10433=ORIENTED_EDGE('',*,*,#7718,.T.) ;
#10434=ORIENTED_EDGE('',*,*,#7724,.T.) ;
#10435=ORIENTED_EDGE('',*,*,#7720,.T.) ;
#10436=ORIENTED_EDGE('',*,*,#7723,.T.) ;
#10437=ORIENTED_EDGE('',*,*,#7725,.T.) ;
#10438=ORIENTED_EDGE('',*,*,#7726,.F.) ;
#10439=ORIENTED_EDGE('',*,*,#7727,.F.) ;
#10440=ORIENTED_EDGE('',*,*,#7728,.F.) ;
#10441=ORIENTED_EDGE('',*,*,#7725,.F.) ;
#10442=ORIENTED_EDGE('',*,*,#7729,.F.) ;
#10443=ORIENTED_EDGE('',*,*,#7730,.T.) ;
#10444=ORIENTED_EDGE('',*,*,#7731,.T.) ;
#10445=ORIENTED_EDGE('',*,*,#7732,.F.) ;
#10446=ORIENTED_EDGE('',*,*,#7726,.T.) ;
#10447=ORIENTED_EDGE('',*,*,#7728,.T.) ;
#10448=ORIENTED_EDGE('',*,*,#7733,.F.) ;
#10449=ORIENTED_EDGE('',*,*,#7734,.T.) ;
#10450=ORIENTED_EDGE('',*,*,#7684,.F.) ;
#10451=ORIENTED_EDGE('',*,*,#7735,.F.) ;
#10452=ORIENTED_EDGE('',*,*,#7685,.F.) ;
#10453=ORIENTED_EDGE('',*,*,#7734,.F.) ;
#10454=ORIENTED_EDGE('',*,*,#7736,.F.) ;
#10455=ORIENTED_EDGE('',*,*,#7735,.T.) ;
#10456=ORIENTED_EDGE('',*,*,#7687,.F.) ;
#10457=ORIENTED_EDGE('',*,*,#7737,.T.) ;
#10458=ORIENTED_EDGE('',*,*,#7688,.F.) ;
#10459=ORIENTED_EDGE('',*,*,#7738,.F.) ;
#10460=ORIENTED_EDGE('',*,*,#7689,.F.) ;
#10461=ORIENTED_EDGE('',*,*,#7737,.F.) ;
#10462=ORIENTED_EDGE('',*,*,#7686,.F.) ;
#10463=ORIENTED_EDGE('',*,*,#7738,.T.) ;
#10464=ORIENTED_EDGE('',*,*,#7691,.F.) ;
#10465=ORIENTED_EDGE('',*,*,#7739,.T.) ;
#10466=ORIENTED_EDGE('',*,*,#7740,.F.) ;
#10467=ORIENTED_EDGE('',*,*,#7741,.F.) ;
#10468=ORIENTED_EDGE('',*,*,#7742,.F.) ;
#10469=ORIENTED_EDGE('',*,*,#7739,.F.) ;
#10470=ORIENTED_EDGE('',*,*,#7690,.F.) ;
#10471=ORIENTED_EDGE('',*,*,#7741,.T.) ;
#10472=ORIENTED_EDGE('',*,*,#7743,.F.) ;
#10473=ORIENTED_EDGE('',*,*,#7744,.T.) ;
#10474=ORIENTED_EDGE('',*,*,#7745,.F.) ;
#10475=ORIENTED_EDGE('',*,*,#7746,.F.) ;
#10476=ORIENTED_EDGE('',*,*,#7747,.F.) ;
#10477=ORIENTED_EDGE('',*,*,#7744,.F.) ;
#10478=ORIENTED_EDGE('',*,*,#7748,.F.) ;
#10479=ORIENTED_EDGE('',*,*,#7746,.T.) ;
#10480=ORIENTED_EDGE('',*,*,#7749,.F.) ;
#10481=ORIENTED_EDGE('',*,*,#7750,.T.) ;
#10482=ORIENTED_EDGE('',*,*,#7692,.F.) ;
#10483=ORIENTED_EDGE('',*,*,#7751,.F.) ;
#10484=ORIENTED_EDGE('',*,*,#7693,.F.) ;
#10485=ORIENTED_EDGE('',*,*,#7750,.F.) ;
#10486=ORIENTED_EDGE('',*,*,#7752,.F.) ;
#10487=ORIENTED_EDGE('',*,*,#7751,.T.) ;
#10488=ORIENTED_EDGE('',*,*,#7695,.F.) ;
#10489=ORIENTED_EDGE('',*,*,#7753,.T.) ;
#10490=ORIENTED_EDGE('',*,*,#7696,.F.) ;
#10491=ORIENTED_EDGE('',*,*,#7754,.F.) ;
#10492=ORIENTED_EDGE('',*,*,#7697,.F.) ;
#10493=ORIENTED_EDGE('',*,*,#7753,.F.) ;
#10494=ORIENTED_EDGE('',*,*,#7694,.F.) ;
#10495=ORIENTED_EDGE('',*,*,#7754,.T.) ;
#10496=ORIENTED_EDGE('',*,*,#7699,.F.) ;
#10497=ORIENTED_EDGE('',*,*,#7755,.T.) ;
#10498=ORIENTED_EDGE('',*,*,#7756,.F.) ;
#10499=ORIENTED_EDGE('',*,*,#7757,.F.) ;
#10500=ORIENTED_EDGE('',*,*,#7758,.F.) ;
#10501=ORIENTED_EDGE('',*,*,#7755,.F.) ;
#10502=ORIENTED_EDGE('',*,*,#7698,.F.) ;
#10503=ORIENTED_EDGE('',*,*,#7757,.T.) ;
#10504=ORIENTED_EDGE('',*,*,#7759,.F.) ;
#10505=ORIENTED_EDGE('',*,*,#7760,.T.) ;
#10506=ORIENTED_EDGE('',*,*,#7761,.F.) ;
#10507=ORIENTED_EDGE('',*,*,#7762,.F.) ;
#10508=ORIENTED_EDGE('',*,*,#7763,.F.) ;
#10509=ORIENTED_EDGE('',*,*,#7760,.F.) ;
#10510=ORIENTED_EDGE('',*,*,#7764,.F.) ;
#10511=ORIENTED_EDGE('',*,*,#7762,.T.) ;
#10512=ORIENTED_EDGE('',*,*,#7765,.F.) ;
#10513=ORIENTED_EDGE('',*,*,#7766,.T.) ;
#10514=ORIENTED_EDGE('',*,*,#7700,.F.) ;
#10515=ORIENTED_EDGE('',*,*,#7767,.F.) ;
#10516=ORIENTED_EDGE('',*,*,#7701,.F.) ;
#10517=ORIENTED_EDGE('',*,*,#7766,.F.) ;
#10518=ORIENTED_EDGE('',*,*,#7768,.F.) ;
#10519=ORIENTED_EDGE('',*,*,#7767,.T.) ;
#10520=ORIENTED_EDGE('',*,*,#7703,.F.) ;
#10521=ORIENTED_EDGE('',*,*,#7769,.T.) ;
#10522=ORIENTED_EDGE('',*,*,#7704,.F.) ;
#10523=ORIENTED_EDGE('',*,*,#7770,.F.) ;
#10524=ORIENTED_EDGE('',*,*,#7705,.F.) ;
#10525=ORIENTED_EDGE('',*,*,#7769,.F.) ;
#10526=ORIENTED_EDGE('',*,*,#7702,.F.) ;
#10527=ORIENTED_EDGE('',*,*,#7770,.T.) ;
#10528=ORIENTED_EDGE('',*,*,#7707,.F.) ;
#10529=ORIENTED_EDGE('',*,*,#7771,.T.) ;
#10530=ORIENTED_EDGE('',*,*,#7772,.F.) ;
#10531=ORIENTED_EDGE('',*,*,#7773,.F.) ;
#10532=ORIENTED_EDGE('',*,*,#7774,.F.) ;
#10533=ORIENTED_EDGE('',*,*,#7771,.F.) ;
#10534=ORIENTED_EDGE('',*,*,#7706,.F.) ;
#10535=ORIENTED_EDGE('',*,*,#7773,.T.) ;
#10536=ORIENTED_EDGE('',*,*,#7775,.F.) ;
#10537=ORIENTED_EDGE('',*,*,#7776,.T.) ;
#10538=ORIENTED_EDGE('',*,*,#7777,.F.) ;
#10539=ORIENTED_EDGE('',*,*,#7778,.F.) ;
#10540=ORIENTED_EDGE('',*,*,#7779,.F.) ;
#10541=ORIENTED_EDGE('',*,*,#7776,.F.) ;
#10542=ORIENTED_EDGE('',*,*,#7780,.F.) ;
#10543=ORIENTED_EDGE('',*,*,#7778,.T.) ;
#10544=ORIENTED_EDGE('',*,*,#7781,.F.) ;
#10545=ORIENTED_EDGE('',*,*,#7782,.T.) ;
#10546=ORIENTED_EDGE('',*,*,#7712,.F.) ;
#10547=ORIENTED_EDGE('',*,*,#7710,.F.) ;
#10548=ORIENTED_EDGE('',*,*,#7783,.F.) ;
#10549=ORIENTED_EDGE('',*,*,#7784,.F.) ;
#10550=ORIENTED_EDGE('',*,*,#7782,.F.) ;
#10551=ORIENTED_EDGE('',*,*,#7785,.F.) ;
#10552=ORIENTED_EDGE('',*,*,#7717,.F.) ;
#10553=ORIENTED_EDGE('',*,*,#7708,.F.) ;
#10554=ORIENTED_EDGE('',*,*,#7716,.F.) ;
#10555=ORIENTED_EDGE('',*,*,#7784,.T.) ;
#10556=ORIENTED_EDGE('',*,*,#7786,.T.) ;
#10557=ORIENTED_EDGE('',*,*,#7787,.F.) ;
#10558=ORIENTED_EDGE('',*,*,#7786,.F.) ;
#10559=ORIENTED_EDGE('',*,*,#7783,.T.) ;
#10560=ORIENTED_EDGE('',*,*,#7713,.F.) ;
#10561=ORIENTED_EDGE('',*,*,#7787,.T.) ;
#10562=ORIENTED_EDGE('',*,*,#7714,.T.) ;
#10563=ORIENTED_EDGE('',*,*,#7785,.T.) ;
#10564=ORIENTED_EDGE('',*,*,#7781,.T.) ;
#10565=ORIENTED_EDGE('',*,*,#7777,.T.) ;
#10566=ORIENTED_EDGE('',*,*,#7779,.T.) ;
#10567=ORIENTED_EDGE('',*,*,#7780,.T.) ;
#10568=ORIENTED_EDGE('',*,*,#7775,.T.) ;
#10569=ORIENTED_EDGE('',*,*,#7772,.T.) ;
#10570=ORIENTED_EDGE('',*,*,#7774,.T.) ;
#10571=ORIENTED_EDGE('',*,*,#7768,.T.) ;
#10572=ORIENTED_EDGE('',*,*,#7765,.T.) ;
#10573=ORIENTED_EDGE('',*,*,#7761,.T.) ;
#10574=ORIENTED_EDGE('',*,*,#7763,.T.) ;
#10575=ORIENTED_EDGE('',*,*,#7764,.T.) ;
#10576=ORIENTED_EDGE('',*,*,#7759,.T.) ;
#10577=ORIENTED_EDGE('',*,*,#7756,.T.) ;
#10578=ORIENTED_EDGE('',*,*,#7758,.T.) ;
#10579=ORIENTED_EDGE('',*,*,#7752,.T.) ;
#10580=ORIENTED_EDGE('',*,*,#7749,.T.) ;
#10581=ORIENTED_EDGE('',*,*,#7745,.T.) ;
#10582=ORIENTED_EDGE('',*,*,#7747,.T.) ;
#10583=ORIENTED_EDGE('',*,*,#7748,.T.) ;
#10584=ORIENTED_EDGE('',*,*,#7743,.T.) ;
#10585=ORIENTED_EDGE('',*,*,#7740,.T.) ;
#10586=ORIENTED_EDGE('',*,*,#7742,.T.) ;
#10587=ORIENTED_EDGE('',*,*,#7736,.T.) ;
#10588=ORIENTED_EDGE('',*,*,#7788,.T.) ;
#10589=ORIENTED_EDGE('',*,*,#7788,.F.) ;
#10590=ORIENTED_EDGE('',*,*,#7733,.T.) ;
#10591=ORIENTED_EDGE('',*,*,#7727,.T.) ;
#10592=ORIENTED_EDGE('',*,*,#7789,.T.) ;
#10593=ORIENTED_EDGE('',*,*,#7731,.F.) ;
#10594=ORIENTED_EDGE('',*,*,#7790,.T.) ;
#10595=ORIENTED_EDGE('',*,*,#7724,.F.) ;
#10596=ORIENTED_EDGE('',*,*,#7790,.F.) ;
#10597=ORIENTED_EDGE('',*,*,#7730,.F.) ;
#10598=ORIENTED_EDGE('',*,*,#7729,.T.) ;
#10599=ORIENTED_EDGE('',*,*,#7722,.T.) ;
#10600=ORIENTED_EDGE('',*,*,#7791,.F.) ;
#10601=ORIENTED_EDGE('',*,*,#7791,.T.) ;
#10602=ORIENTED_EDGE('',*,*,#7721,.T.) ;
#10603=ORIENTED_EDGE('',*,*,#7732,.T.) ;
#10604=ORIENTED_EDGE('',*,*,#7789,.F.) ;
#10605=ORIENTED_EDGE('',*,*,#7792,.F.) ;
#10606=ORIENTED_EDGE('',*,*,#7792,.T.) ;
#10607=ORIENTED_EDGE('',*,*,#7793,.F.) ;
#10608=ORIENTED_EDGE('',*,*,#7793,.T.) ;
#10609=ORIENTED_EDGE('',*,*,#7794,.F.) ;
#10610=ORIENTED_EDGE('',*,*,#7795,.T.) ;
#10611=ORIENTED_EDGE('',*,*,#7795,.F.) ;
#10612=ORIENTED_EDGE('',*,*,#7794,.T.) ;
#10613=ORIENTED_EDGE('',*,*,#7796,.F.) ;
#10614=ORIENTED_EDGE('',*,*,#7796,.T.) ;
#10615=ORIENTED_EDGE('',*,*,#7797,.F.) ;
#10616=ORIENTED_EDGE('',*,*,#7798,.T.) ;
#10617=ORIENTED_EDGE('',*,*,#7798,.F.) ;
#10618=ORIENTED_EDGE('',*,*,#7797,.T.) ;
#10619=ORIENTED_EDGE('',*,*,#7799,.F.) ;
#10620=ORIENTED_EDGE('',*,*,#7799,.T.) ;
#10621=ORIENTED_EDGE('',*,*,#7800,.F.) ;
#10622=ORIENTED_EDGE('',*,*,#7801,.T.) ;
#10623=ORIENTED_EDGE('',*,*,#7801,.F.) ;
#10624=ORIENTED_EDGE('',*,*,#7800,.T.) ;
#10625=ORIENTED_EDGE('',*,*,#7802,.F.) ;
#10626=ORIENTED_EDGE('',*,*,#7802,.T.) ;
#10627=ORIENTED_EDGE('',*,*,#7803,.F.) ;
#10628=ORIENTED_EDGE('',*,*,#7804,.T.) ;
#10629=ORIENTED_EDGE('',*,*,#7804,.F.) ;
#10630=ORIENTED_EDGE('',*,*,#7803,.T.) ;
#10631=ORIENTED_EDGE('',*,*,#7805,.F.) ;
#10632=ORIENTED_EDGE('',*,*,#7805,.T.) ;
#12150=PLANE('',#14697) ;
#12151=PLANE('',#14762) ;
#12704=ADVANCED_FACE('',(#3309),#390,.F.) ;
#12705=ADVANCED_FACE('',(#3310),#391,.T.) ;
#12706=ADVANCED_FACE('',(#3311),#392,.F.) ;
#12707=ADVANCED_FACE('',(#3312),#393,.F.) ;
#12708=ADVANCED_FACE('',(#3313),#394,.F.) ;
#12709=ADVANCED_FACE('',(#3314),#2844,.F.) ;
#12710=ADVANCED_FACE('',(#3315),#395,.T.) ;
#12711=ADVANCED_FACE('',(#3316),#396,.T.) ;
#12712=ADVANCED_FACE('',(#3317),#397,.F.) ;
#12713=ADVANCED_FACE('',(#3318),#398,.T.) ;
#12714=ADVANCED_FACE('',(#3319),#2845,.T.) ;
#12715=ADVANCED_FACE('',(#3320),#399,.F.) ;
#12716=ADVANCED_FACE('',(#3321),#400,.T.) ;
#12717=ADVANCED_FACE('',(#3322),#401,.T.) ;
#12718=ADVANCED_FACE('',(#3323),#402,.F.) ;
#12719=ADVANCED_FACE('',(#3324),#403,.F.) ;
#12720=ADVANCED_FACE('',(#3325),#404,.T.) ;
#12721=ADVANCED_FACE('',(#3326),#405,.F.) ;
#12722=ADVANCED_FACE('',(#3327),#406,.T.) ;
#12723=ADVANCED_FACE('',(#3328),#407,.F.) ;
#12724=ADVANCED_FACE('',(#3329),#408,.T.) ;
#12725=ADVANCED_FACE('',(#3330),#409,.T.) ;
#12726=ADVANCED_FACE('',(#3331),#410,.F.) ;
#12727=ADVANCED_FACE('',(#3332),#411,.F.) ;
#12728=ADVANCED_FACE('',(#3333),#412,.T.) ;
#12729=ADVANCED_FACE('',(#3334),#413,.F.) ;
#12730=ADVANCED_FACE('',(#3335),#414,.T.) ;
#12731=ADVANCED_FACE('',(#3336),#415,.F.) ;
#12732=ADVANCED_FACE('',(#3337),#416,.T.) ;
#12733=ADVANCED_FACE('',(#3338),#417,.T.) ;
#12734=ADVANCED_FACE('',(#3339),#418,.F.) ;
#12735=ADVANCED_FACE('',(#3340),#419,.F.) ;
#12736=ADVANCED_FACE('',(#3341),#420,.T.) ;
#12737=ADVANCED_FACE('',(#3342),#421,.F.) ;
#12738=ADVANCED_FACE('',(#3343),#422,.T.) ;
#12739=ADVANCED_FACE('',(#3344),#423,.F.) ;
#12740=ADVANCED_FACE('',(#3345),#424,.T.) ;
#12741=ADVANCED_FACE('',(#3346),#425,.T.) ;
#12742=ADVANCED_FACE('',(#3347),#426,.F.) ;
#12743=ADVANCED_FACE('',(#3348),#427,.F.) ;
#12744=ADVANCED_FACE('',(#3349),#428,.T.) ;
#12745=ADVANCED_FACE('',(#3350),#429,.F.) ;
#12746=ADVANCED_FACE('',(#3351),#430,.T.) ;
#12747=ADVANCED_FACE('',(#3352,#857),#431,.F.) ;
#12748=ADVANCED_FACE('',(#3353),#432,.T.) ;
#12749=ADVANCED_FACE('',(#3354),#433,.T.) ;
#12750=ADVANCED_FACE('',(#3355),#434,.F.) ;
#12751=ADVANCED_FACE('',(#3356),#435,.F.) ;
#12752=ADVANCED_FACE('',(#3357),#436,.T.) ;
#12753=ADVANCED_FACE('',(#3358,#858),#437,.F.) ;
#12754=ADVANCED_FACE('',(#3359),#438,.T.) ;
#12755=ADVANCED_FACE('',(#3360,#859),#439,.F.) ;
#12756=ADVANCED_FACE('',(#3361),#440,.T.) ;
#12757=ADVANCED_FACE('',(#3362),#441,.T.) ;
#12758=ADVANCED_FACE('',(#3363),#442,.F.) ;
#12759=ADVANCED_FACE('',(#3364),#443,.F.) ;
#12760=ADVANCED_FACE('',(#3365),#444,.T.) ;
#12761=ADVANCED_FACE('',(#3366),#2846,.F.) ;
#12762=ADVANCED_FACE('',(#3367),#445,.F.) ;
#12763=ADVANCED_FACE('',(#3368),#446,.F.) ;
#12764=ADVANCED_FACE('',(#3369),#447,.F.) ;
#12765=ADVANCED_FACE('',(#3370),#448,.T.) ;
#12766=ADVANCED_FACE('',(#3371),#449,.F.) ;
#12767=ADVANCED_FACE('',(#3372),#450,.T.) ;
#12768=ADVANCED_FACE('',(#3373,#860),#451,.F.) ;
#12769=ADVANCED_FACE('',(#3374),#2847,.T.) ;
#12770=ADVANCED_FACE('',(#3375),#452,.T.) ;
#12771=ADVANCED_FACE('',(#3376),#453,.T.) ;
#12772=ADVANCED_FACE('',(#3377),#454,.T.) ;
#12773=ADVANCED_FACE('',(#3378),#455,.T.) ;
#12774=ADVANCED_FACE('',(#3379),#456,.T.) ;
#12775=ADVANCED_FACE('',(#3380),#457,.T.) ;
#12776=ADVANCED_FACE('',(#3381),#458,.T.) ;
#12777=ADVANCED_FACE('',(#3382),#459,.T.) ;
#12778=ADVANCED_FACE('',(#3383),#460,.T.) ;
#12779=ADVANCED_FACE('',(#3384),#2848,.F.) ;
#12780=ADVANCED_FACE('',(#3385),#2849,.T.) ;
#12781=ADVANCED_FACE('',(#3386,#861),#12150,.T.) ;
#12782=ADVANCED_FACE('',(#3387),#2850,.T.) ;
#12783=ADVANCED_FACE('',(#3388),#2851,.T.) ;
#12784=ADVANCED_FACE('',(#3389),#2852,.T.) ;
#12785=ADVANCED_FACE('',(#3390),#2853,.T.) ;
#12786=ADVANCED_FACE('',(#3391),#2854,.T.) ;
#12787=ADVANCED_FACE('',(#3392),#2855,.T.) ;
#12788=ADVANCED_FACE('',(#3393),#2856,.T.) ;
#12789=ADVANCED_FACE('',(#3394),#2857,.T.) ;
#12790=ADVANCED_FACE('',(#3395),#2858,.T.) ;
#12791=ADVANCED_FACE('',(#3396),#2859,.T.) ;
#12792=ADVANCED_FACE('',(#3397),#2860,.T.) ;
#12793=ADVANCED_FACE('',(#3398),#2861,.T.) ;
#12794=ADVANCED_FACE('',(#3399),#2862,.T.) ;
#12795=ADVANCED_FACE('',(#3400),#2863,.T.) ;
#12796=ADVANCED_FACE('',(#3401),#2864,.T.) ;
#12797=ADVANCED_FACE('',(#3402),#2865,.T.) ;
#12798=ADVANCED_FACE('',(#3403),#2866,.T.) ;
#12799=ADVANCED_FACE('',(#3404,#862),#12151,.T.) ;
#12800=ADVANCED_FACE('',(#3405),#461,.T.) ;
#12801=ADVANCED_FACE('',(#3406),#462,.T.) ;
#12802=ADVANCED_FACE('',(#3407),#463,.T.) ;
#12803=ADVANCED_FACE('',(#3408),#464,.T.) ;
#12804=ADVANCED_FACE('',(#3409),#465,.T.) ;
#12805=ADVANCED_FACE('',(#3410),#466,.T.) ;
#12806=ADVANCED_FACE('',(#3411),#467,.T.) ;
#12807=ADVANCED_FACE('',(#3412),#2867,.F.) ;
#12808=ADVANCED_FACE('',(#3413),#468,.T.) ;
#12809=ADVANCED_FACE('',(#3414),#469,.T.) ;
#12810=ADVANCED_FACE('',(#3415),#470,.F.) ;
#12811=ADVANCED_FACE('',(#3416),#471,.F.) ;
#12812=ADVANCED_FACE('',(#3417),#472,.F.) ;
#12813=ADVANCED_FACE('',(#3418),#473,.F.) ;
#12814=ADVANCED_FACE('',(#3419),#474,.F.) ;
#12815=ADVANCED_FACE('',(#3420),#475,.F.) ;
#12816=ADVANCED_FACE('',(#3421),#476,.F.) ;
#12817=ADVANCED_FACE('',(#3422),#477,.F.) ;
#12818=ADVANCED_FACE('',(#3423),#478,.F.) ;
#12819=ADVANCED_FACE('',(#3424),#479,.F.) ;
#12820=ADVANCED_FACE('',(#3425),#480,.F.) ;
#12821=ADVANCED_FACE('',(#3426),#481,.F.) ;
#13133=CLOSED_SHELL('',(#12704,#12705)) ;
#13134=CLOSED_SHELL('',(#12706,#12707)) ;
#13135=CLOSED_SHELL('',(#12708,#12709,#12710)) ;
#13136=CLOSED_SHELL('',(#12711,#12712,#12713,#12714)) ;
#13137=CLOSED_SHELL('',(#12715,#12716,#12717)) ;
#13138=CLOSED_SHELL('',(#12718,#12719)) ;
#13139=CLOSED_SHELL('',(#12720,#12721,#12722)) ;
#13140=CLOSED_SHELL('',(#12723,#12724,#12725)) ;
#13141=CLOSED_SHELL('',(#12726,#12727)) ;
#13142=CLOSED_SHELL('',(#12728,#12729,#12730)) ;
#13143=CLOSED_SHELL('',(#12731,#12732,#12733)) ;
#13144=CLOSED_SHELL('',(#12734,#12735)) ;
#13145=CLOSED_SHELL('',(#12736,#12737,#12738)) ;
#13146=CLOSED_SHELL('',(#12739,#12740,#12741)) ;
#13147=CLOSED_SHELL('',(#12742,#12743)) ;
#13148=CLOSED_SHELL('',(#12744,#12745,#12746)) ;
#13149=CLOSED_SHELL('',(#12747,#12748,#12749)) ;
#13150=CLOSED_SHELL('',(#12750,#12751)) ;
#13151=CLOSED_SHELL('',(#12752,#12753,#12754)) ;
#13152=CLOSED_SHELL('',(#12755,#12756,#12757)) ;
#13153=CLOSED_SHELL('',(#12758,#12759)) ;
#13154=CLOSED_SHELL('',(#12760,#12761,#12762)) ;
#13155=CLOSED_SHELL('',(#12763,#12764)) ;
#13156=CLOSED_SHELL('',(#12765,#12766)) ;
#13157=CLOSED_SHELL('',(#12767,#12768,#12769,#12770)) ;
#13158=CLOSED_SHELL('',(#12771,#12772,#12773,#12774,#12775,#12776,#12777,
#12778,#12779,#12780,#12781,#12782,#12783,#12784,#12785,#12786,#12787,#12788,
#12789,#12790,#12791,#12792,#12793,#12794,#12795,#12796,#12797,#12798,#12799,
#12800,#12801,#12802,#12803,#12804,#12805,#12806,#12807,#12808,#12809)) ;
#13159=CLOSED_SHELL('',(#12810,#12811)) ;
#13160=CLOSED_SHELL('',(#12812,#12813)) ;
#13161=CLOSED_SHELL('',(#12814,#12815)) ;
#13162=CLOSED_SHELL('',(#12816,#12817)) ;
#13163=CLOSED_SHELL('',(#12818,#12819)) ;
#13164=CLOSED_SHELL('',(#12820,#12821)) ;
#14495=AXIS2_PLACEMENT_3D('',#21616,#17463,#17464) ;
#14496=AXIS2_PLACEMENT_3D('',#21617,#17465,#17466) ;
#14497=AXIS2_PLACEMENT_3D('',#21619,#17467,#17468) ;
#14498=AXIS2_PLACEMENT_3D('',#21621,#17469,#17470) ;
#14499=AXIS2_PLACEMENT_3D('',#21622,#17471,#17472) ;
#14500=AXIS2_PLACEMENT_3D('',#21624,#17473,#17474) ;
#14501=AXIS2_PLACEMENT_3D('',#21625,#17475,#17476) ;
#14502=AXIS2_PLACEMENT_3D('',#21627,#17477,#17478) ;
#14503=AXIS2_PLACEMENT_3D('',#21629,#17479,#17480) ;
#14504=AXIS2_PLACEMENT_3D('',#21630,#17481,#17482) ;
#14505=AXIS2_PLACEMENT_3D('',#21632,#17483,#17484) ;
#14506=AXIS2_PLACEMENT_3D('',#21633,#17485,#17486) ;
#14507=AXIS2_PLACEMENT_3D('',#21636,#17487,#17488) ;
#14508=AXIS2_PLACEMENT_3D('',#21651,#17489,#17490) ;
#14509=AXIS2_PLACEMENT_3D('',#21652,#17491,#17492) ;
#14510=AXIS2_PLACEMENT_3D('',#21653,#17493,#17494) ;
#14511=AXIS2_PLACEMENT_3D('',#21654,#17495,#17496) ;
#14512=AXIS2_PLACEMENT_3D('',#21656,#17497,#17498) ;
#14513=AXIS2_PLACEMENT_3D('',#21658,#17499,#17500) ;
#14514=AXIS2_PLACEMENT_3D('',#21659,#17501,#17502) ;
#14515=AXIS2_PLACEMENT_3D('',#21661,#17503,#17504) ;
#14516=AXIS2_PLACEMENT_3D('',#21689,#17505,#17506) ;
#14517=AXIS2_PLACEMENT_3D('',#21690,#17507,#17508) ;
#14518=AXIS2_PLACEMENT_3D('',#21691,#17509,#17510) ;
#14519=AXIS2_PLACEMENT_3D('',#21692,#17511,#17512) ;
#14520=AXIS2_PLACEMENT_3D('',#21693,#17513,#17514) ;
#14521=AXIS2_PLACEMENT_3D('',#21695,#17515,#17516) ;
#14522=AXIS2_PLACEMENT_3D('',#21697,#17517,#17518) ;
#14523=AXIS2_PLACEMENT_3D('',#21698,#17519,#17520) ;
#14524=AXIS2_PLACEMENT_3D('',#21699,#17521,#17522) ;
#14525=AXIS2_PLACEMENT_3D('',#21701,#17523,#17524) ;
#14526=AXIS2_PLACEMENT_3D('',#21702,#17525,#17526) ;
#14527=AXIS2_PLACEMENT_3D('',#21704,#17527,#17528) ;
#14528=AXIS2_PLACEMENT_3D('',#21705,#17529,#17530) ;
#14529=AXIS2_PLACEMENT_3D('',#21707,#17531,#17532) ;
#14530=AXIS2_PLACEMENT_3D('',#21709,#17533,#17534) ;
#14531=AXIS2_PLACEMENT_3D('',#21710,#17535,#17536) ;
#14532=AXIS2_PLACEMENT_3D('',#21712,#17537,#17538) ;
#14533=AXIS2_PLACEMENT_3D('',#21713,#17539,#17540) ;
#14534=AXIS2_PLACEMENT_3D('',#21715,#17541,#17542) ;
#14535=AXIS2_PLACEMENT_3D('',#21717,#17543,#17544) ;
#14536=AXIS2_PLACEMENT_3D('',#21718,#17545,#17546) ;
#14537=AXIS2_PLACEMENT_3D('',#21720,#17547,#17548) ;
#14538=AXIS2_PLACEMENT_3D('',#21721,#17549,#17550) ;
#14539=AXIS2_PLACEMENT_3D('',#21722,#17551,#17552) ;
#14540=AXIS2_PLACEMENT_3D('',#21724,#17553,#17554) ;
#14541=AXIS2_PLACEMENT_3D('',#21725,#17555,#17556) ;
#14542=AXIS2_PLACEMENT_3D('',#21727,#17557,#17558) ;
#14543=AXIS2_PLACEMENT_3D('',#21729,#17559,#17560) ;
#14544=AXIS2_PLACEMENT_3D('',#21730,#17561,#17562) ;
#14545=AXIS2_PLACEMENT_3D('',#21731,#17563,#17564) ;
#14546=AXIS2_PLACEMENT_3D('',#21733,#17565,#17566) ;
#14547=AXIS2_PLACEMENT_3D('',#21734,#17567,#17568) ;
#14548=AXIS2_PLACEMENT_3D('',#21736,#17569,#17570) ;
#14549=AXIS2_PLACEMENT_3D('',#21737,#17571,#17572) ;
#14550=AXIS2_PLACEMENT_3D('',#21739,#17573,#17574) ;
#14551=AXIS2_PLACEMENT_3D('',#21741,#17575,#17576) ;
#14552=AXIS2_PLACEMENT_3D('',#21742,#17577,#17578) ;
#14553=AXIS2_PLACEMENT_3D('',#21744,#17579,#17580) ;
#14554=AXIS2_PLACEMENT_3D('',#21745,#17581,#17582) ;
#14555=AXIS2_PLACEMENT_3D('',#21747,#17583,#17584) ;
#14556=AXIS2_PLACEMENT_3D('',#21749,#17585,#17586) ;
#14557=AXIS2_PLACEMENT_3D('',#21750,#17587,#17588) ;
#14558=AXIS2_PLACEMENT_3D('',#21752,#17589,#17590) ;
#14559=AXIS2_PLACEMENT_3D('',#21753,#17591,#17592) ;
#14560=AXIS2_PLACEMENT_3D('',#21754,#17593,#17594) ;
#14561=AXIS2_PLACEMENT_3D('',#21756,#17595,#17596) ;
#14562=AXIS2_PLACEMENT_3D('',#21757,#17597,#17598) ;
#14563=AXIS2_PLACEMENT_3D('',#21759,#17599,#17600) ;
#14564=AXIS2_PLACEMENT_3D('',#21761,#17601,#17602) ;
#14565=AXIS2_PLACEMENT_3D('',#21762,#17603,#17604) ;
#14566=AXIS2_PLACEMENT_3D('',#21763,#17605,#17606) ;
#14567=AXIS2_PLACEMENT_3D('',#21765,#17607,#17608) ;
#14568=AXIS2_PLACEMENT_3D('',#21766,#17609,#17610) ;
#14569=AXIS2_PLACEMENT_3D('',#21768,#17611,#17612) ;
#14570=AXIS2_PLACEMENT_3D('',#21769,#17613,#17614) ;
#14571=AXIS2_PLACEMENT_3D('',#21771,#17615,#17616) ;
#14572=AXIS2_PLACEMENT_3D('',#21773,#17617,#17618) ;
#14573=AXIS2_PLACEMENT_3D('',#21774,#17619,#17620) ;
#14574=AXIS2_PLACEMENT_3D('',#21776,#17621,#17622) ;
#14575=AXIS2_PLACEMENT_3D('',#21777,#17623,#17624) ;
#14576=AXIS2_PLACEMENT_3D('',#21779,#17625,#17626) ;
#14577=AXIS2_PLACEMENT_3D('',#21781,#17627,#17628) ;
#14578=AXIS2_PLACEMENT_3D('',#21782,#17629,#17630) ;
#14579=AXIS2_PLACEMENT_3D('',#21784,#17631,#17632) ;
#14580=AXIS2_PLACEMENT_3D('',#21785,#17633,#17634) ;
#14581=AXIS2_PLACEMENT_3D('',#21786,#17635,#17636) ;
#14582=AXIS2_PLACEMENT_3D('',#21788,#17637,#17638) ;
#14583=AXIS2_PLACEMENT_3D('',#21789,#17639,#17640) ;
#14584=AXIS2_PLACEMENT_3D('',#21791,#17641,#17642) ;
#14585=AXIS2_PLACEMENT_3D('',#21793,#17643,#17644) ;
#14586=AXIS2_PLACEMENT_3D('',#21794,#17645,#17646) ;
#14587=AXIS2_PLACEMENT_3D('',#21795,#17647,#17648) ;
#14588=AXIS2_PLACEMENT_3D('',#21797,#17649,#17650) ;
#14589=AXIS2_PLACEMENT_3D('',#21798,#17651,#17652) ;
#14590=AXIS2_PLACEMENT_3D('',#21799,#17653,#17654) ;
#14591=AXIS2_PLACEMENT_3D('',#21801,#17655,#17656) ;
#14592=AXIS2_PLACEMENT_3D('',#21802,#17657,#17658) ;
#14593=AXIS2_PLACEMENT_3D('',#21803,#17659,#17660) ;
#14594=AXIS2_PLACEMENT_3D('',#21805,#17661,#17662) ;
#14595=AXIS2_PLACEMENT_3D('',#21806,#17663,#17664) ;
#14596=AXIS2_PLACEMENT_3D('',#21808,#17665,#17666) ;
#14597=AXIS2_PLACEMENT_3D('',#21809,#17667,#17668) ;
#14598=AXIS2_PLACEMENT_3D('',#21810,#17669,#17670) ;
#14599=AXIS2_PLACEMENT_3D('',#21811,#17671,#17672) ;
#14600=AXIS2_PLACEMENT_3D('',#21813,#17673,#17674) ;
#14601=AXIS2_PLACEMENT_3D('',#21815,#17675,#17676) ;
#14602=AXIS2_PLACEMENT_3D('',#21817,#17677,#17678) ;
#14603=AXIS2_PLACEMENT_3D('',#21818,#17679,#17680) ;
#14604=AXIS2_PLACEMENT_3D('',#21819,#17681,#17682) ;
#14605=AXIS2_PLACEMENT_3D('',#21820,#17683,#17684) ;
#14606=AXIS2_PLACEMENT_3D('',#21822,#17685,#17686) ;
#14607=AXIS2_PLACEMENT_3D('',#21823,#17687,#17688) ;
#14608=AXIS2_PLACEMENT_3D('',#21824,#17689,#17690) ;
#14609=AXIS2_PLACEMENT_3D('',#21826,#17691,#17692) ;
#14610=AXIS2_PLACEMENT_3D('',#21827,#17693,#17694) ;
#14611=AXIS2_PLACEMENT_3D('',#21830,#17695,#17696) ;
#14612=AXIS2_PLACEMENT_3D('',#21832,#17697,#17698) ;
#14613=AXIS2_PLACEMENT_3D('',#21833,#17699,#17700) ;
#14614=AXIS2_PLACEMENT_3D('',#21835,#17701,#17702) ;
#14615=AXIS2_PLACEMENT_3D('',#21836,#17703,#17704) ;
#14616=AXIS2_PLACEMENT_3D('',#21837,#17705,#17706) ;
#14617=AXIS2_PLACEMENT_3D('',#21840,#17707,#17708) ;
#14618=AXIS2_PLACEMENT_3D('',#21842,#17709,#17710) ;
#14619=AXIS2_PLACEMENT_3D('',#21843,#17711,#17712) ;
#14620=AXIS2_PLACEMENT_3D('',#21845,#17713,#17714) ;
#14621=AXIS2_PLACEMENT_3D('',#21847,#17715,#17716) ;
#14622=AXIS2_PLACEMENT_3D('',#21848,#17717,#17718) ;
#14623=AXIS2_PLACEMENT_3D('',#21849,#17719,#17720) ;
#14624=AXIS2_PLACEMENT_3D('',#21850,#17721,#17722) ;
#14625=AXIS2_PLACEMENT_3D('',#21852,#17723,#17724) ;
#14626=AXIS2_PLACEMENT_3D('',#21853,#17725,#17726) ;
#14627=AXIS2_PLACEMENT_3D('',#21854,#17727,#17728) ;
#14628=AXIS2_PLACEMENT_3D('',#21857,#17729,#17730) ;
#14629=AXIS2_PLACEMENT_3D('',#21858,#17731,#17732) ;
#14630=AXIS2_PLACEMENT_3D('',#21859,#17733,#17734) ;
#14631=AXIS2_PLACEMENT_3D('',#21870,#17735,#17736) ;
#14632=AXIS2_PLACEMENT_3D('',#21871,#17737,#17738) ;
#14633=AXIS2_PLACEMENT_3D('',#21873,#17739,#17740) ;
#14634=AXIS2_PLACEMENT_3D('',#21874,#17741,#17742) ;
#14635=AXIS2_PLACEMENT_3D('',#21875,#17743,#17744) ;
#14636=AXIS2_PLACEMENT_3D('',#21878,#17745,#17746) ;
#14637=AXIS2_PLACEMENT_3D('',#21879,#17747,#17748) ;
#14638=AXIS2_PLACEMENT_3D('',#21880,#17749,#17750) ;
#14639=AXIS2_PLACEMENT_3D('',#21882,#17751,#17752) ;
#14640=AXIS2_PLACEMENT_3D('',#21884,#17753,#17754) ;
#14641=AXIS2_PLACEMENT_3D('',#21885,#17755,#17756) ;
#14642=AXIS2_PLACEMENT_3D('',#21888,#17757,#17758) ;
#14643=AXIS2_PLACEMENT_3D('',#21889,#17759,#17760) ;
#14644=AXIS2_PLACEMENT_3D('',#21890,#17761,#17762) ;
#14645=AXIS2_PLACEMENT_3D('',#21893,#17763,#17764) ;
#14646=AXIS2_PLACEMENT_3D('',#21895,#17765,#17766) ;
#14647=AXIS2_PLACEMENT_3D('',#21896,#17767,#17768) ;
#14648=AXIS2_PLACEMENT_3D('',#21898,#17769,#17770) ;
#14649=AXIS2_PLACEMENT_3D('',#21921,#17771,#17772) ;
#14650=AXIS2_PLACEMENT_3D('',#21922,#17773,#17774) ;
#14651=AXIS2_PLACEMENT_3D('',#21923,#17775,#17776) ;
#14652=AXIS2_PLACEMENT_3D('',#21926,#17777,#17778) ;
#14653=AXIS2_PLACEMENT_3D('',#21928,#17779,#17780) ;
#14654=AXIS2_PLACEMENT_3D('',#21930,#17781,#17782) ;
#14655=AXIS2_PLACEMENT_3D('',#21931,#17783,#17784) ;
#14656=AXIS2_PLACEMENT_3D('',#21932,#17785,#17786) ;
#14657=AXIS2_PLACEMENT_3D('',#21935,#17787,#17788) ;
#14658=AXIS2_PLACEMENT_3D('',#21937,#17789,#17790) ;
#14659=AXIS2_PLACEMENT_3D('',#21939,#17791,#17792) ;
#14660=AXIS2_PLACEMENT_3D('',#21940,#17793,#17794) ;
#14661=AXIS2_PLACEMENT_3D('',#21941,#17795,#17796) ;
#14662=AXIS2_PLACEMENT_3D('',#21944,#17797,#17798) ;
#14663=AXIS2_PLACEMENT_3D('',#21946,#17799,#17800) ;
#14664=AXIS2_PLACEMENT_3D('',#21948,#17801,#17802) ;
#14665=AXIS2_PLACEMENT_3D('',#21949,#17803,#17804) ;
#14666=AXIS2_PLACEMENT_3D('',#21950,#17805,#17806) ;
#14667=AXIS2_PLACEMENT_3D('',#21953,#17807,#17808) ;
#14668=AXIS2_PLACEMENT_3D('',#21955,#17809,#17810) ;
#14669=AXIS2_PLACEMENT_3D('',#21957,#17811,#17812) ;
#14670=AXIS2_PLACEMENT_3D('',#21958,#17813,#17814) ;
#14671=AXIS2_PLACEMENT_3D('',#21959,#17815,#17816) ;
#14672=AXIS2_PLACEMENT_3D('',#21962,#17817,#17818) ;
#14673=AXIS2_PLACEMENT_3D('',#21964,#17819,#17820) ;
#14674=AXIS2_PLACEMENT_3D('',#21966,#17821,#17822) ;
#14675=AXIS2_PLACEMENT_3D('',#21967,#17823,#17824) ;
#14676=AXIS2_PLACEMENT_3D('',#21968,#17825,#17826) ;
#14677=AXIS2_PLACEMENT_3D('',#21971,#17827,#17828) ;
#14678=AXIS2_PLACEMENT_3D('',#21973,#17829,#17830) ;
#14679=AXIS2_PLACEMENT_3D('',#21975,#17831,#17832) ;
#14680=AXIS2_PLACEMENT_3D('',#21976,#17833,#17834) ;
#14681=AXIS2_PLACEMENT_3D('',#21977,#17835,#17836) ;
#14682=AXIS2_PLACEMENT_3D('',#21980,#17837,#17838) ;
#14683=AXIS2_PLACEMENT_3D('',#21981,#17839,#17840) ;
#14684=AXIS2_PLACEMENT_3D('',#21982,#17841,#17842) ;
#14685=AXIS2_PLACEMENT_3D('',#21985,#17843,#17844) ;
#14686=AXIS2_PLACEMENT_3D('',#21987,#17845,#17846) ;
#14687=AXIS2_PLACEMENT_3D('',#21989,#17847,#17848) ;
#14688=AXIS2_PLACEMENT_3D('',#21990,#17849,#17850) ;
#14689=AXIS2_PLACEMENT_3D('',#21991,#17851,#17852) ;
#14690=AXIS2_PLACEMENT_3D('',#21993,#17853,#17854) ;
#14691=AXIS2_PLACEMENT_3D('',#22026,#17856,#17857) ;
#14692=AXIS2_PLACEMENT_3D('',#22028,#17858,#17859) ;
#14693=AXIS2_PLACEMENT_3D('',#22032,#17861,#17862) ;
#14694=AXIS2_PLACEMENT_3D('',#22034,#17863,#17864) ;
#14695=AXIS2_PLACEMENT_3D('',#22036,#17865,#17866) ;
#14696=AXIS2_PLACEMENT_3D('',#22037,#17867,#17868) ;
#14697=AXIS2_PLACEMENT_3D('',#22038,#17869,#17870) ;
#14698=AXIS2_PLACEMENT_3D('',#22040,#17871,#17872) ;
#14699=AXIS2_PLACEMENT_3D('',#22041,#17873,#17874) ;
#14700=AXIS2_PLACEMENT_3D('',#22045,#17876,#17877) ;
#14701=AXIS2_PLACEMENT_3D('',#22047,#17878,#17879) ;
#14702=AXIS2_PLACEMENT_3D('',#22048,#17880,#17881) ;
#14703=AXIS2_PLACEMENT_3D('',#22049,#17882,#17883) ;
#14704=AXIS2_PLACEMENT_3D('',#22050,#17884,#17885) ;
#14705=AXIS2_PLACEMENT_3D('',#22084,#17886,#17887) ;
#14706=AXIS2_PLACEMENT_3D('',#22085,#17888,#17889) ;
#14707=AXIS2_PLACEMENT_3D('',#22087,#17890,#17891) ;
#14708=AXIS2_PLACEMENT_3D('',#22089,#17893,#17894) ;
#14709=AXIS2_PLACEMENT_3D('',#22090,#17895,#17896) ;
#14710=AXIS2_PLACEMENT_3D('',#22091,#17897,#17898) ;
#14711=AXIS2_PLACEMENT_3D('',#22093,#17900,#17901) ;
#14712=AXIS2_PLACEMENT_3D('',#22094,#17902,#17903) ;
#14713=AXIS2_PLACEMENT_3D('',#22098,#17905,#17906) ;
#14714=AXIS2_PLACEMENT_3D('',#22100,#17907,#17908) ;
#14715=AXIS2_PLACEMENT_3D('',#22101,#17909,#17910) ;
#14716=AXIS2_PLACEMENT_3D('',#22102,#17911,#17912) ;
#14717=AXIS2_PLACEMENT_3D('',#22104,#17913,#17914) ;
#14718=AXIS2_PLACEMENT_3D('',#22108,#17916,#17917) ;
#14719=AXIS2_PLACEMENT_3D('',#22110,#17918,#17919) ;
#14720=AXIS2_PLACEMENT_3D('',#22111,#17920,#17921) ;
#14721=AXIS2_PLACEMENT_3D('',#22112,#17922,#17923) ;
#14722=AXIS2_PLACEMENT_3D('',#22113,#17924,#17925) ;
#14723=AXIS2_PLACEMENT_3D('',#22115,#17926,#17927) ;
#14724=AXIS2_PLACEMENT_3D('',#22117,#17929,#17930) ;
#14725=AXIS2_PLACEMENT_3D('',#22118,#17931,#17932) ;
#14726=AXIS2_PLACEMENT_3D('',#22119,#17933,#17934) ;
#14727=AXIS2_PLACEMENT_3D('',#22121,#17936,#17937) ;
#14728=AXIS2_PLACEMENT_3D('',#22122,#17938,#17939) ;
#14729=AXIS2_PLACEMENT_3D('',#22126,#17941,#17942) ;
#14730=AXIS2_PLACEMENT_3D('',#22128,#17943,#17944) ;
#14731=AXIS2_PLACEMENT_3D('',#22129,#17945,#17946) ;
#14732=AXIS2_PLACEMENT_3D('',#22130,#17947,#17948) ;
#14733=AXIS2_PLACEMENT_3D('',#22132,#17949,#17950) ;
#14734=AXIS2_PLACEMENT_3D('',#22136,#17952,#17953) ;
#14735=AXIS2_PLACEMENT_3D('',#22138,#17954,#17955) ;
#14736=AXIS2_PLACEMENT_3D('',#22139,#17956,#17957) ;
#14737=AXIS2_PLACEMENT_3D('',#22140,#17958,#17959) ;
#14738=AXIS2_PLACEMENT_3D('',#22141,#17960,#17961) ;
#14739=AXIS2_PLACEMENT_3D('',#22143,#17962,#17963) ;
#14740=AXIS2_PLACEMENT_3D('',#22145,#17965,#17966) ;
#14741=AXIS2_PLACEMENT_3D('',#22146,#17967,#17968) ;
#14742=AXIS2_PLACEMENT_3D('',#22147,#17969,#17970) ;
#14743=AXIS2_PLACEMENT_3D('',#22149,#17972,#17973) ;
#14744=AXIS2_PLACEMENT_3D('',#22150,#17974,#17975) ;
#14745=AXIS2_PLACEMENT_3D('',#22154,#17977,#17978) ;
#14746=AXIS2_PLACEMENT_3D('',#22156,#17979,#17980) ;
#14747=AXIS2_PLACEMENT_3D('',#22157,#17981,#17982) ;
#14748=AXIS2_PLACEMENT_3D('',#22158,#17983,#17984) ;
#14749=AXIS2_PLACEMENT_3D('',#22160,#17985,#17986) ;
#14750=AXIS2_PLACEMENT_3D('',#22164,#17988,#17989) ;
#14751=AXIS2_PLACEMENT_3D('',#22166,#17990,#17991) ;
#14752=AXIS2_PLACEMENT_3D('',#22167,#17992,#17993) ;
#14753=AXIS2_PLACEMENT_3D('',#22168,#17994,#17995) ;
#14754=AXIS2_PLACEMENT_3D('',#22169,#17996,#17997) ;
#14755=AXIS2_PLACEMENT_3D('',#22171,#17998,#17999) ;
#14756=AXIS2_PLACEMENT_3D('',#22174,#18001,#18002) ;
#14757=AXIS2_PLACEMENT_3D('',#22175,#18003,#18004) ;
#14758=AXIS2_PLACEMENT_3D('',#22176,#18005,#18006) ;
#14759=AXIS2_PLACEMENT_3D('',#22177,#18007,#18008) ;
#14760=AXIS2_PLACEMENT_3D('',#22178,#18009,#18010) ;
#14761=AXIS2_PLACEMENT_3D('',#22181,#18012,#18013) ;
#14762=AXIS2_PLACEMENT_3D('',#22182,#18014,#18015) ;
#14763=AXIS2_PLACEMENT_3D('',#22183,#18016,#18017) ;
#14764=AXIS2_PLACEMENT_3D('',#22184,#18018,#18019) ;
#14765=AXIS2_PLACEMENT_3D('',#22185,#18020,#18021) ;
#14766=AXIS2_PLACEMENT_3D('',#22186,#18022,#18023) ;
#14767=AXIS2_PLACEMENT_3D('',#22187,#18024,#18025) ;
#14768=AXIS2_PLACEMENT_3D('',#22188,#18026,#18027) ;
#14769=AXIS2_PLACEMENT_3D('',#22189,#18028,#18029) ;
#14770=AXIS2_PLACEMENT_3D('',#22191,#18030,#18031) ;
#14771=AXIS2_PLACEMENT_3D('',#22192,#18032,#18033) ;
#14772=AXIS2_PLACEMENT_3D('',#22193,#18034,#18035) ;
#14773=AXIS2_PLACEMENT_3D('',#22195,#18037,#18038) ;
#14774=AXIS2_PLACEMENT_3D('',#22197,#18039,#18040) ;
#14775=AXIS2_PLACEMENT_3D('',#22198,#18041,#18042) ;
#14776=AXIS2_PLACEMENT_3D('',#22199,#18043,#18044) ;
#14777=AXIS2_PLACEMENT_3D('',#22201,#18045,#18046) ;
#14778=AXIS2_PLACEMENT_3D('',#22202,#18047,#18048) ;
#14779=AXIS2_PLACEMENT_3D('',#22203,#18049,#18050) ;
#14780=AXIS2_PLACEMENT_3D('',#22205,#18051,#18052) ;
#14781=AXIS2_PLACEMENT_3D('',#22206,#18053,#18054) ;
#14782=AXIS2_PLACEMENT_3D('',#22207,#18055,#18056) ;
#14783=AXIS2_PLACEMENT_3D('',#22209,#18057,#18058) ;
#14784=AXIS2_PLACEMENT_3D('',#22211,#18059,#18060) ;
#14785=AXIS2_PLACEMENT_3D('',#22212,#18061,#18062) ;
#14786=AXIS2_PLACEMENT_3D('',#22214,#18063,#18064) ;
#14787=AXIS2_PLACEMENT_3D('',#22215,#18065,#18066) ;
#14788=AXIS2_PLACEMENT_3D('',#22217,#18067,#18068) ;
#14789=AXIS2_PLACEMENT_3D('',#22219,#18069,#18070) ;
#14790=AXIS2_PLACEMENT_3D('',#22220,#18071,#18072) ;
#14791=AXIS2_PLACEMENT_3D('',#22222,#18073,#18074) ;
#14792=AXIS2_PLACEMENT_3D('',#22223,#18075,#18076) ;
#14793=AXIS2_PLACEMENT_3D('',#22225,#18077,#18078) ;
#14794=AXIS2_PLACEMENT_3D('',#22227,#18079,#18080) ;
#14795=AXIS2_PLACEMENT_3D('',#22228,#18081,#18082) ;
#14796=AXIS2_PLACEMENT_3D('',#22230,#18083,#18084) ;
#14797=AXIS2_PLACEMENT_3D('',#22231,#18085,#18086) ;
#14798=AXIS2_PLACEMENT_3D('',#22233,#18087,#18088) ;
#14799=AXIS2_PLACEMENT_3D('',#22235,#18089,#18090) ;
#14800=AXIS2_PLACEMENT_3D('',#22236,#18091,#18092) ;
#14801=AXIS2_PLACEMENT_3D('',#22238,#18093,#18094) ;
#17463=DIRECTION('axis',(0.,0.,1.)) ;
#17464=DIRECTION('refdir',(1.,0.,0.)) ;
#17465=DIRECTION('center_axis',(0.,0.,1.)) ;
#17466=DIRECTION('ref_axis',(1.,0.,0.)) ;
#17467=DIRECTION('center_axis',(-0.350791170819065,0.,-0.936453711870154)) ;
#17468=DIRECTION('ref_axis',(0.,-1.,0.)) ;
#17469=DIRECTION('center_axis',(0.,1.,0.)) ;
#17470=DIRECTION('ref_axis',(-1.,0.,0.)) ;
#17471=DIRECTION('center_axis',(0.,0.,1.)) ;
#17472=DIRECTION('ref_axis',(1.,0.,0.)) ;
#17473=DIRECTION('center_axis',(0.,-1.,0.)) ;
#17474=DIRECTION('ref_axis',(-1.,0.,0.)) ;
#17475=DIRECTION('center_axis',(0.,0.,1.)) ;
#17476=DIRECTION('ref_axis',(1.,0.,0.)) ;
#17477=DIRECTION('center_axis',(0.350791170819065,0.,0.936453711870154)) ;
#17478=DIRECTION('ref_axis',(0.,1.,0.)) ;
#17479=DIRECTION('center_axis',(0.,1.,0.)) ;
#17480=DIRECTION('ref_axis',(-1.,0.,0.)) ;
#17481=DIRECTION('center_axis',(0.,0.,1.)) ;
#17482=DIRECTION('ref_axis',(1.,0.,0.)) ;
#17483=DIRECTION('center_axis',(0.,1.,0.)) ;
#17484=DIRECTION('ref_axis',(-1.,0.,0.)) ;
#17485=DIRECTION('center_axis',(0.,0.,1.)) ;
#17486=DIRECTION('ref_axis',(1.,0.,0.)) ;
#17487=DIRECTION('center_axis',(-0.350791170819065,0.,-0.936453711870154)) ;
#17488=DIRECTION('ref_axis',(0.,-1.,0.)) ;
#17489=DIRECTION('center_axis',(0.,1.,0.)) ;
#17490=DIRECTION('ref_axis',(1.,0.,0.)) ;
#17491=DIRECTION('center_axis',(0.,1.,0.)) ;
#17492=DIRECTION('ref_axis',(1.,0.,0.)) ;
#17493=DIRECTION('center_axis',(0.,0.,1.)) ;
#17494=DIRECTION('ref_axis',(1.,0.,0.)) ;
#17495=DIRECTION('center_axis',(0.,0.,1.)) ;
#17496=DIRECTION('ref_axis',(1.,0.,0.)) ;
#17497=DIRECTION('center_axis',(-0.201200039678648,0.,-0.979550174331724)) ;
#17498=DIRECTION('ref_axis',(0.,-1.,0.)) ;
#17499=DIRECTION('center_axis',(0.,-1.,0.)) ;
#17500=DIRECTION('ref_axis',(-1.,0.,0.)) ;
#17501=DIRECTION('center_axis',(0.,0.,1.)) ;
#17502=DIRECTION('ref_axis',(1.,0.,0.)) ;
#17503=DIRECTION('center_axis',(0.,1.,0.)) ;
#17504=DIRECTION('ref_axis',(-1.,0.,0.)) ;
#17505=DIRECTION('center_axis',(-0.350791170819065,0.,-0.936453711870154)) ;
#17506=DIRECTION('ref_axis',(0.,-1.,0.)) ;
#17507=DIRECTION('center_axis',(1.,0.,0.)) ;
#17508=DIRECTION('ref_axis',(0.,-1.,0.)) ;
#17509=DIRECTION('center_axis',(0.,1.,0.)) ;
#17510=DIRECTION('ref_axis',(1.,0.,0.)) ;
#17511=DIRECTION('center_axis',(0.,1.,0.)) ;
#17512=DIRECTION('ref_axis',(1.,0.,0.)) ;
#17513=DIRECTION('center_axis',(0.,0.,1.)) ;
#17514=DIRECTION('ref_axis',(1.,0.,0.)) ;
#17515=DIRECTION('center_axis',(-0.0467328634842026,0.,-0.998907422872894)) ;
#17516=DIRECTION('ref_axis',(0.,-1.,0.)) ;
#17517=DIRECTION('center_axis',(0.,1.,0.)) ;
#17518=DIRECTION('ref_axis',(-1.,0.,0.)) ;
#17519=DIRECTION('center_axis',(-0.201200039678648,0.,-0.979550174331724)) ;
#17520=DIRECTION('ref_axis',(0.,-1.,0.)) ;
#17521=DIRECTION('center_axis',(0.,0.,1.)) ;
#17522=DIRECTION('ref_axis',(1.,0.,0.)) ;
#17523=DIRECTION('center_axis',(0.,-1.,0.)) ;
#17524=DIRECTION('ref_axis',(-1.,0.,0.)) ;
#17525=DIRECTION('center_axis',(0.,0.,1.)) ;
#17526=DIRECTION('ref_axis',(1.,0.,0.)) ;
#17527=DIRECTION('center_axis',(0.,-1.,0.)) ;
#17528=DIRECTION('ref_axis',(-1.,0.,0.)) ;
#17529=DIRECTION('center_axis',(0.,0.,1.)) ;
#17530=DIRECTION('ref_axis',(1.,0.,0.)) ;
#17531=DIRECTION('center_axis',(0.0467328634842026,0.,0.998907422872894)) ;
#17532=DIRECTION('ref_axis',(0.,1.,0.)) ;
#17533=DIRECTION('center_axis',(0.,1.,0.)) ;
#17534=DIRECTION('ref_axis',(-1.,0.,0.)) ;
#17535=DIRECTION('center_axis',(0.,0.,1.)) ;
#17536=DIRECTION('ref_axis',(1.,0.,0.)) ;
#17537=DIRECTION('center_axis',(0.,1.,0.)) ;
#17538=DIRECTION('ref_axis',(-1.,0.,0.)) ;
#17539=DIRECTION('center_axis',(0.,0.,1.)) ;
#17540=DIRECTION('ref_axis',(1.,0.,0.)) ;
#17541=DIRECTION('center_axis',(0.108866874851964,0.,-0.99405633822232)) ;
#17542=DIRECTION('ref_axis',(0.,-1.,0.)) ;
#17543=DIRECTION('center_axis',(0.,-1.,0.)) ;
#17544=DIRECTION('ref_axis',(-1.,0.,0.)) ;
#17545=DIRECTION('center_axis',(0.,0.,1.)) ;
#17546=DIRECTION('ref_axis',(1.,0.,0.)) ;
#17547=DIRECTION('center_axis',(0.,1.,0.)) ;
#17548=DIRECTION('ref_axis',(-1.,0.,0.)) ;
#17549=DIRECTION('center_axis',(-0.0467328634842026,0.,-0.998907422872894)) ;
#17550=DIRECTION('ref_axis',(0.,-1.,0.)) ;
#17551=DIRECTION('center_axis',(0.,0.,1.)) ;
#17552=DIRECTION('ref_axis',(1.,0.,0.)) ;
#17553=DIRECTION('center_axis',(0.,-1.,0.)) ;
#17554=DIRECTION('ref_axis',(-1.,0.,0.)) ;
#17555=DIRECTION('center_axis',(0.,0.,1.)) ;
#17556=DIRECTION('ref_axis',(1.,0.,0.)) ;
#17557=DIRECTION('center_axis',(0.261828244987421,0.,-0.965114485502527)) ;
#17558=DIRECTION('ref_axis',(0.,-1.,0.)) ;
#17559=DIRECTION('center_axis',(0.,1.,0.)) ;
#17560=DIRECTION('ref_axis',(-1.,0.,0.)) ;
#17561=DIRECTION('center_axis',(0.108866874851964,0.,-0.99405633822232)) ;
#17562=DIRECTION('ref_axis',(0.,-1.,0.)) ;
#17563=DIRECTION('center_axis',(0.,0.,1.)) ;
#17564=DIRECTION('ref_axis',(1.,0.,0.)) ;
#17565=DIRECTION('center_axis',(0.,-1.,0.)) ;
#17566=DIRECTION('ref_axis',(-1.,0.,0.)) ;
#17567=DIRECTION('center_axis',(0.,0.,1.)) ;
#17568=DIRECTION('ref_axis',(1.,0.,0.)) ;
#17569=DIRECTION('center_axis',(0.,-1.,0.)) ;
#17570=DIRECTION('ref_axis',(-1.,0.,0.)) ;
#17571=DIRECTION('center_axis',(0.,0.,1.)) ;
#17572=DIRECTION('ref_axis',(1.,0.,0.)) ;
#17573=DIRECTION('center_axis',(-0.261828244987421,0.,0.965114485502527)) ;
#17574=DIRECTION('ref_axis',(0.,1.,0.)) ;
#17575=DIRECTION('center_axis',(0.,1.,0.)) ;
#17576=DIRECTION('ref_axis',(-1.,0.,0.)) ;
#17577=DIRECTION('center_axis',(0.,0.,1.)) ;
#17578=DIRECTION('ref_axis',(1.,0.,0.)) ;
#17579=DIRECTION('center_axis',(0.,1.,0.)) ;
#17580=DIRECTION('ref_axis',(-1.,0.,0.)) ;
#17581=DIRECTION('center_axis',(0.,0.,1.)) ;
#17582=DIRECTION('ref_axis',(1.,0.,0.)) ;
#17583=DIRECTION('center_axis',(0.408444256935997,0.,-0.912783265061319)) ;
#17584=DIRECTION('ref_axis',(0.,-1.,0.)) ;
#17585=DIRECTION('center_axis',(0.,-1.,0.)) ;
#17586=DIRECTION('ref_axis',(-1.,0.,0.)) ;
#17587=DIRECTION('center_axis',(0.,0.,1.)) ;
#17588=DIRECTION('ref_axis',(1.,0.,0.)) ;
#17589=DIRECTION('center_axis',(0.,1.,0.)) ;
#17590=DIRECTION('ref_axis',(-1.,0.,0.)) ;
#17591=DIRECTION('center_axis',(0.261828244987421,0.,-0.965114485502527)) ;
#17592=DIRECTION('ref_axis',(0.,-1.,0.)) ;
#17593=DIRECTION('center_axis',(0.,0.,1.)) ;
#17594=DIRECTION('ref_axis',(1.,0.,0.)) ;
#17595=DIRECTION('center_axis',(0.,-1.,0.)) ;
#17596=DIRECTION('ref_axis',(-1.,0.,0.)) ;
#17597=DIRECTION('center_axis',(0.,0.,1.)) ;
#17598=DIRECTION('ref_axis',(1.,0.,0.)) ;
#17599=DIRECTION('center_axis',(0.545161699271658,0.,-0.838330914166499)) ;
#17600=DIRECTION('ref_axis',(0.,-1.,0.)) ;
#17601=DIRECTION('center_axis',(0.,1.,0.)) ;
#17602=DIRECTION('ref_axis',(-1.,0.,0.)) ;
#17603=DIRECTION('center_axis',(0.408444256935997,0.,-0.912783265061319)) ;
#17604=DIRECTION('ref_axis',(0.,-1.,0.)) ;
#17605=DIRECTION('center_axis',(0.,0.,1.)) ;
#17606=DIRECTION('ref_axis',(1.,0.,0.)) ;
#17607=DIRECTION('center_axis',(0.,-1.,0.)) ;
#17608=DIRECTION('ref_axis',(-1.,0.,0.)) ;
#17609=DIRECTION('center_axis',(0.,0.,1.)) ;
#17610=DIRECTION('ref_axis',(1.,0.,0.)) ;
#17611=DIRECTION('center_axis',(0.,-1.,0.)) ;
#17612=DIRECTION('ref_axis',(-1.,0.,0.)) ;
#17613=DIRECTION('center_axis',(0.,0.,1.)) ;
#17614=DIRECTION('ref_axis',(1.,0.,0.)) ;
#17615=DIRECTION('center_axis',(-0.545161699271658,0.,0.838330914166499)) ;
#17616=DIRECTION('ref_axis',(0.,1.,0.)) ;
#17617=DIRECTION('center_axis',(0.,1.,0.)) ;
#17618=DIRECTION('ref_axis',(-1.,0.,0.)) ;
#17619=DIRECTION('center_axis',(0.,0.,1.)) ;
#17620=DIRECTION('ref_axis',(1.,0.,0.)) ;
#17621=DIRECTION('center_axis',(0.,1.,0.)) ;
#17622=DIRECTION('ref_axis',(-1.,0.,0.)) ;
#17623=DIRECTION('center_axis',(0.,0.,1.)) ;
#17624=DIRECTION('ref_axis',(1.,0.,0.)) ;
#17625=DIRECTION('center_axis',(0.668667250537987,0.,-0.743561771514626)) ;
#17626=DIRECTION('ref_axis',(0.,-1.,0.)) ;
#17627=DIRECTION('center_axis',(0.,-1.,0.)) ;
#17628=DIRECTION('ref_axis',(-1.,0.,0.)) ;
#17629=DIRECTION('center_axis',(0.,0.,1.)) ;
#17630=DIRECTION('ref_axis',(1.,0.,0.)) ;
#17631=DIRECTION('center_axis',(0.,1.,0.)) ;
#17632=DIRECTION('ref_axis',(-1.,0.,0.)) ;
#17633=DIRECTION('center_axis',(0.545161699271658,0.,-0.838330914166499)) ;
#17634=DIRECTION('ref_axis',(0.,-1.,0.)) ;
#17635=DIRECTION('center_axis',(0.,0.,1.)) ;
#17636=DIRECTION('ref_axis',(1.,0.,0.)) ;
#17637=DIRECTION('center_axis',(0.,-1.,0.)) ;
#17638=DIRECTION('ref_axis',(-1.,0.,0.)) ;
#17639=DIRECTION('center_axis',(0.,0.,1.)) ;
#17640=DIRECTION('ref_axis',(1.,0.,0.)) ;
#17641=DIRECTION('center_axis',(0.775967776969404,0.,-0.630772549422659)) ;
#17642=DIRECTION('ref_axis',(0.,-1.,0.)) ;
#17643=DIRECTION('center_axis',(0.,1.,0.)) ;
#17644=DIRECTION('ref_axis',(-1.,0.,0.)) ;
#17645=DIRECTION('center_axis',(0.668667250537987,0.,-0.743561771514626)) ;
#17646=DIRECTION('ref_axis',(0.,-1.,0.)) ;
#17647=DIRECTION('center_axis',(0.,0.,1.)) ;
#17648=DIRECTION('ref_axis',(1.,0.,0.)) ;
#17649=DIRECTION('center_axis',(0.,-1.,0.)) ;
#17650=DIRECTION('ref_axis',(-1.,0.,0.)) ;
#17651=DIRECTION('center_axis',(0.,0.,1.)) ;
#17652=DIRECTION('ref_axis',(-0.999997170842168,0.00237871975216741,0.)) ;
#17653=DIRECTION('center_axis',(0.,0.,1.)) ;
#17654=DIRECTION('ref_axis',(1.,0.,0.)) ;
#17655=DIRECTION('center_axis',(-0.775967776969404,0.,0.630772549422659)) ;
#17656=DIRECTION('ref_axis',(0.,1.,0.)) ;
#17657=DIRECTION('center_axis',(0.,0.,1.)) ;
#17658=DIRECTION('ref_axis',(-0.999996539011801,-0.00263096264124049,0.)) ;
#17659=DIRECTION('center_axis',(0.,0.,1.)) ;
#17660=DIRECTION('ref_axis',(-0.999994323348501,-0.00336946149617212,0.)) ;
#17661=DIRECTION('center_axis',(0.864462870524064,0.,-0.502696673437666)) ;
#17662=DIRECTION('ref_axis',(0.,-1.,0.)) ;
#17663=DIRECTION('center_axis',(0.,0.,1.)) ;
#17664=DIRECTION('ref_axis',(1.,0.,0.)) ;
#17665=DIRECTION('center_axis',(0.,1.,0.)) ;
#17666=DIRECTION('ref_axis',(-1.,0.,0.)) ;
#17667=DIRECTION('center_axis',(0.775967776969404,0.,-0.630772549422659)) ;
#17668=DIRECTION('ref_axis',(0.,-1.,0.)) ;
#17669=DIRECTION('center_axis',(0.,0.,1.)) ;
#17670=DIRECTION('ref_axis',(1.,0.,0.)) ;
#17671=DIRECTION('center_axis',(0.,0.,1.)) ;
#17672=DIRECTION('ref_axis',(1.,0.,0.)) ;
#17673=DIRECTION('center_axis',(0.864462870524064,0.,-0.502696673437666)) ;
#17674=DIRECTION('ref_axis',(0.,-1.,0.)) ;
#17675=DIRECTION('center_axis',(0.,1.,0.)) ;
#17676=DIRECTION('ref_axis',(-1.,0.,0.)) ;
#17677=DIRECTION('center_axis',(0.932007869282798,0.,-0.362438038283702)) ;
#17678=DIRECTION('ref_axis',(0.362438038283702,0.,0.932007869282798)) ;
#17679=DIRECTION('center_axis',(0.,0.,1.)) ;
#17680=DIRECTION('ref_axis',(1.,0.,0.)) ;
#17681=DIRECTION('center_axis',(0.,0.,1.)) ;
#17682=DIRECTION('ref_axis',(-0.999991061612965,-0.00422808398397034,0.)) ;
#17683=DIRECTION('center_axis',(0.,0.,1.)) ;
#17684=DIRECTION('ref_axis',(1.,0.,0.)) ;
#17685=DIRECTION('center_axis',(-0.932007869282798,0.,0.362438038283702)) ;
#17686=DIRECTION('ref_axis',(-0.362438038283702,0.,-0.932007869282798)) ;
#17687=DIRECTION('center_axis',(0.,0.,1.)) ;
#17688=DIRECTION('ref_axis',(-0.99998657479322,0.00518172107739271,0.)) ;
#17689=DIRECTION('center_axis',(0.,0.,1.)) ;
#17690=DIRECTION('ref_axis',(-0.999999956889578,0.000293633856850915,0.)) ;
#17691=DIRECTION('center_axis',(0.976965832926672,0.,-0.213395785557951)) ;
#17692=DIRECTION('ref_axis',(0.213395785557951,0.,0.976965832926672)) ;
#17693=DIRECTION('center_axis',(0.,0.,1.)) ;
#17694=DIRECTION('ref_axis',(1.,0.,0.)) ;
#17695=DIRECTION('center_axis',(0.932007869282798,0.,-0.362438038283702)) ;
#17696=DIRECTION('ref_axis',(0.362438038283702,0.,0.932007869282798)) ;
#17697=DIRECTION('center_axis',(0.,1.,0.)) ;
#17698=DIRECTION('ref_axis',(-1.,0.,0.)) ;
#17699=DIRECTION('center_axis',(0.932007869282798,0.,-0.362438038283702)) ;
#17700=DIRECTION('ref_axis',(0.362438038283702,0.,0.932007869282798)) ;
#17701=DIRECTION('center_axis',(0.,1.,0.)) ;
#17702=DIRECTION('ref_axis',(-1.,0.,0.)) ;
#17703=DIRECTION('center_axis',(0.,0.,1.)) ;
#17704=DIRECTION('ref_axis',(1.,0.,0.)) ;
#17705=DIRECTION('center_axis',(0.,0.,1.)) ;
#17706=DIRECTION('ref_axis',(1.,0.,0.)) ;
#17707=DIRECTION('center_axis',(0.976965832926672,0.,-0.213395785557951)) ;
#17708=DIRECTION('ref_axis',(0.213395785557951,0.,0.976965832926672)) ;
#17709=DIRECTION('center_axis',(0.,1.,0.)) ;
#17710=DIRECTION('ref_axis',(-1.,0.,0.)) ;
#17711=DIRECTION('center_axis',(0.976965832926672,0.,-0.213395785557951)) ;
#17712=DIRECTION('ref_axis',(0.213395785557951,0.,0.976965832926672)) ;
#17713=DIRECTION('center_axis',(0.,1.,0.)) ;
#17714=DIRECTION('ref_axis',(-1.,0.,0.)) ;
#17715=DIRECTION('center_axis',(0.998247213677188,0.,-0.0591819261745526)) ;
#17716=DIRECTION('ref_axis',(0.0591819261745526,0.,0.998247213677188)) ;
#17717=DIRECTION('center_axis',(0.,0.,1.)) ;
#17718=DIRECTION('ref_axis',(1.,0.,0.)) ;
#17719=DIRECTION('center_axis',(-5.94762334620619E-17,0.,1.)) ;
#17720=DIRECTION('ref_axis',(-0.999999583069371,0.000913159944786785,0.)) ;
#17721=DIRECTION('center_axis',(0.,0.,1.)) ;
#17722=DIRECTION('ref_axis',(1.,0.,0.)) ;
#17723=DIRECTION('center_axis',(-0.998247213677188,0.,0.0591819261745526)) ;
#17724=DIRECTION('ref_axis',(-0.0591819261745526,0.,-0.998247213677188)) ;
#17725=DIRECTION('center_axis',(-5.04646829375071E-17,0.,1.)) ;
#17726=DIRECTION('ref_axis',(-0.999999999326038,3.67140843060554E-5,0.)) ;
#17727=DIRECTION('center_axis',(0.,0.,1.)) ;
#17728=DIRECTION('ref_axis',(1.,0.,0.)) ;
#17729=DIRECTION('center_axis',(0.995336261281429,0.,0.0964661960393706)) ;
#17730=DIRECTION('ref_axis',(-0.0964661960393706,0.,0.995336261281429)) ;
#17731=DIRECTION('center_axis',(0.,1.,0.)) ;
#17732=DIRECTION('ref_axis',(1.,0.,0.)) ;
#17733=DIRECTION('center_axis',(0.,-1.,0.)) ;
#17734=DIRECTION('ref_axis',(-0.995336261281429,0.,-0.0964661960393711)) ;
#17735=DIRECTION('center_axis',(5.04646829375071E-17,0.,1.)) ;
#17736=DIRECTION('ref_axis',(1.,0.,0.)) ;
#17737=DIRECTION('center_axis',(0.,0.,1.)) ;
#17738=DIRECTION('ref_axis',(-0.999999839691638,-0.000566230251627689,0.)) ;
#17739=DIRECTION('center_axis',(-0.995336261281429,0.,-0.0964661960393706)) ;
#17740=DIRECTION('ref_axis',(0.0964661960393706,0.,-0.995336261281429)) ;
#17741=DIRECTION('center_axis',(5.04646829375071E-17,0.,1.)) ;
#17742=DIRECTION('ref_axis',(1.,0.,0.)) ;
#17743=DIRECTION('center_axis',(5.94762334620619E-17,0.,1.)) ;
#17744=DIRECTION('ref_axis',(1.,0.,0.)) ;
#17745=DIRECTION('center_axis',(0.995336261281429,0.,0.0964661960393706)) ;
#17746=DIRECTION('ref_axis',(-0.0964661960393706,0.,0.995336261281429)) ;
#17747=DIRECTION('center_axis',(0.995336261281429,0.,0.0964661960393706)) ;
#17748=DIRECTION('ref_axis',(-0.0964661960393706,0.,0.995336261281429)) ;
#17749=DIRECTION('center_axis',(0.,0.,1.)) ;
#17750=DIRECTION('ref_axis',(1.,0.,0.)) ;
#17751=DIRECTION('center_axis',(0.,1.,0.)) ;
#17752=DIRECTION('ref_axis',(-1.,0.,0.)) ;
#17753=DIRECTION('center_axis',(0.,1.,0.)) ;
#17754=DIRECTION('ref_axis',(-1.,0.,0.)) ;
#17755=DIRECTION('center_axis',(0.,0.,1.)) ;
#17756=DIRECTION('ref_axis',(1.,0.,0.)) ;
#17757=DIRECTION('center_axis',(0.995336261281429,0.,0.0964661960393706)) ;
#17758=DIRECTION('ref_axis',(-0.0964661960393706,0.,0.995336261281429)) ;
#17759=DIRECTION('center_axis',(0.,1.,0.)) ;
#17760=DIRECTION('ref_axis',(1.,0.,0.)) ;
#17761=DIRECTION('center_axis',(5.04646829375071E-17,0.,1.)) ;
#17762=DIRECTION('ref_axis',(1.,0.,0.)) ;
#17763=DIRECTION('center_axis',(0.998247213677188,0.,-0.0591819261745526)) ;
#17764=DIRECTION('ref_axis',(0.0591819261745526,0.,0.998247213677188)) ;
#17765=DIRECTION('center_axis',(0.,1.,0.)) ;
#17766=DIRECTION('ref_axis',(-1.,0.,0.)) ;
#17767=DIRECTION('center_axis',(0.998247213677188,0.,-0.0591819261745526)) ;
#17768=DIRECTION('ref_axis',(0.0591819261745526,0.,0.998247213677188)) ;
#17769=DIRECTION('center_axis',(0.,1.,0.)) ;
#17770=DIRECTION('ref_axis',(-1.,0.,0.)) ;
#17771=DIRECTION('center_axis',(0.,-1.,0.)) ;
#17772=DIRECTION('ref_axis',(-0.995336261281429,0.,-0.0964661960393709)) ;
#17773=DIRECTION('center_axis',(0.,0.,1.)) ;
#17774=DIRECTION('ref_axis',(1.,0.,0.)) ;
#17775=DIRECTION('center_axis',(0.,0.,1.)) ;
#17776=DIRECTION('ref_axis',(-1.,0.,0.)) ;
#17777=DIRECTION('center_axis',(-0.998247213677188,0.,0.0591819261745526)) ;
#17778=DIRECTION('ref_axis',(0.0591819261745526,0.,0.998247213677188)) ;
#17779=DIRECTION('center_axis',(-0.998247213677188,0.,0.0591819261745526)) ;
#17780=DIRECTION('ref_axis',(0.0591819261745526,0.,0.998247213677188)) ;
#17781=DIRECTION('center_axis',(0.976965832926672,0.,-0.213395785557951)) ;
#17782=DIRECTION('ref_axis',(0.213395785557951,0.,0.976965832926672)) ;
#17783=DIRECTION('center_axis',(0.976965832926672,0.,-0.213395785557951)) ;
#17784=DIRECTION('ref_axis',(0.213395785557951,0.,0.976965832926672)) ;
#17785=DIRECTION('center_axis',(0.,0.,1.)) ;
#17786=DIRECTION('ref_axis',(-1.,0.,0.)) ;
#17787=DIRECTION('center_axis',(-0.976965832926672,0.,0.213395785557951)) ;
#17788=DIRECTION('ref_axis',(0.213395785557951,0.,0.976965832926672)) ;
#17789=DIRECTION('center_axis',(-0.976965832926672,0.,0.213395785557951)) ;
#17790=DIRECTION('ref_axis',(0.213395785557951,0.,0.976965832926672)) ;
#17791=DIRECTION('center_axis',(0.932007869282798,0.,-0.362438038283702)) ;
#17792=DIRECTION('ref_axis',(0.362438038283702,0.,0.932007869282798)) ;
#17793=DIRECTION('center_axis',(0.932007869282798,0.,-0.362438038283702)) ;
#17794=DIRECTION('ref_axis',(0.362438038283702,0.,0.932007869282798)) ;
#17795=DIRECTION('center_axis',(0.,0.,1.)) ;
#17796=DIRECTION('ref_axis',(-1.,-6.34413156928661E-16,0.)) ;
#17797=DIRECTION('center_axis',(-0.775967776969404,0.,0.630772549422659)) ;
#17798=DIRECTION('ref_axis',(0.630772549422659,0.,0.775967776969404)) ;
#17799=DIRECTION('center_axis',(-0.775967776969404,0.,0.630772549422659)) ;
#17800=DIRECTION('ref_axis',(0.630772549422659,0.,0.775967776969404)) ;
#17801=DIRECTION('center_axis',(0.668667250537987,0.,-0.743561771514626)) ;
#17802=DIRECTION('ref_axis',(0.743561771514626,0.,0.668667250537987)) ;
#17803=DIRECTION('center_axis',(0.668667250537987,0.,-0.743561771514626)) ;
#17804=DIRECTION('ref_axis',(0.743561771514626,0.,0.668667250537987)) ;
#17805=DIRECTION('center_axis',(0.,0.,1.)) ;
#17806=DIRECTION('ref_axis',(-1.,0.,0.)) ;
#17807=DIRECTION('center_axis',(-0.668667250537987,0.,0.743561771514626)) ;
#17808=DIRECTION('ref_axis',(0.743561771514626,0.,0.668667250537987)) ;
#17809=DIRECTION('center_axis',(-0.668667250537987,0.,0.743561771514626)) ;
#17810=DIRECTION('ref_axis',(0.743561771514626,0.,0.668667250537987)) ;
#17811=DIRECTION('center_axis',(0.545161699271658,0.,-0.838330914166499)) ;
#17812=DIRECTION('ref_axis',(0.838330914166499,0.,0.545161699271658)) ;
#17813=DIRECTION('center_axis',(0.545161699271658,0.,-0.838330914166499)) ;
#17814=DIRECTION('ref_axis',(0.838330914166499,0.,0.545161699271658)) ;
#17815=DIRECTION('center_axis',(0.,0.,1.)) ;
#17816=DIRECTION('ref_axis',(-1.,0.,0.)) ;
#17817=DIRECTION('center_axis',(-0.261828244987421,0.,0.965114485502527)) ;
#17818=DIRECTION('ref_axis',(0.965114485502527,0.,0.261828244987421)) ;
#17819=DIRECTION('center_axis',(-0.261828244987421,0.,0.965114485502527)) ;
#17820=DIRECTION('ref_axis',(0.965114485502527,0.,0.261828244987421)) ;
#17821=DIRECTION('center_axis',(0.108866874851964,0.,-0.99405633822232)) ;
#17822=DIRECTION('ref_axis',(0.99405633822232,0.,0.108866874851965)) ;
#17823=DIRECTION('center_axis',(0.108866874851964,0.,-0.99405633822232)) ;
#17824=DIRECTION('ref_axis',(0.99405633822232,0.,0.108866874851965)) ;
#17825=DIRECTION('center_axis',(0.,0.,1.)) ;
#17826=DIRECTION('ref_axis',(-1.,0.,0.)) ;
#17827=DIRECTION('center_axis',(-0.108866874851964,0.,0.99405633822232)) ;
#17828=DIRECTION('ref_axis',(0.99405633822232,0.,0.108866874851965)) ;
#17829=DIRECTION('center_axis',(-0.108866874851964,0.,0.99405633822232)) ;
#17830=DIRECTION('ref_axis',(0.99405633822232,0.,0.108866874851965)) ;
#17831=DIRECTION('center_axis',(-0.0467328634842026,0.,-0.998907422872894)) ;
#17832=DIRECTION('ref_axis',(0.998907422872894,0.,-0.0467328634842026)) ;
#17833=DIRECTION('center_axis',(-0.0467328634842026,0.,-0.998907422872894)) ;
#17834=DIRECTION('ref_axis',(0.998907422872894,0.,-0.0467328634842026)) ;
#17835=DIRECTION('center_axis',(0.,0.,1.)) ;
#17836=DIRECTION('ref_axis',(1.,0.,0.)) ;
#17837=DIRECTION('center_axis',(0.350791170819065,0.,0.936453711870154)) ;
#17838=DIRECTION('ref_axis',(0.936453711870154,0.,-0.350791170819065)) ;
#17839=DIRECTION('center_axis',(0.,1.,0.)) ;
#17840=DIRECTION('ref_axis',(1.,0.,0.)) ;
#17841=DIRECTION('center_axis',(0.577350269189626,0.577350269189626,0.577350269189626)) ;
#17842=DIRECTION('ref_axis',(-0.707106781186548,0.,0.707106781186548)) ;
#17843=DIRECTION('center_axis',(0.350791170819065,0.,0.936453711870154)) ;
#17844=DIRECTION('ref_axis',(0.936453711870154,0.,-0.350791170819065)) ;
#17845=DIRECTION('center_axis',(-0.408248290463863,0.816496580927726,-0.408248290463863)) ;
#17846=DIRECTION('ref_axis',(0.707106781186548,0.,-0.707106781186548)) ;
#17847=DIRECTION('center_axis',(0.350791170819065,0.,0.936453711870154)) ;
#17848=DIRECTION('ref_axis',(0.936453711870154,0.,-0.350791170819065)) ;
#17849=DIRECTION('center_axis',(0.,1.,0.)) ;
#17850=DIRECTION('ref_axis',(1.,0.,0.)) ;
#17851=DIRECTION('center_axis',(0.,1.,0.)) ;
#17852=DIRECTION('ref_axis',(1.,0.,0.)) ;
#17853=DIRECTION('center_axis',(0.,1.,0.)) ;
#17854=DIRECTION('ref_axis',(1.,0.,0.)) ;
#17855=DIRECTION('',(0.,1.,0.)) ;
#17856=DIRECTION('center_axis',(0.,-1.,0.)) ;
#17857=DIRECTION('ref_axis',(1.,0.,0.)) ;
#17858=DIRECTION('center_axis',(0.,-1.,0.)) ;
#17859=DIRECTION('ref_axis',(1.,0.,0.)) ;
#17860=DIRECTION('',(0.,1.,0.)) ;
#17861=DIRECTION('center_axis',(-0.703809019912964,0.707106781186547,-0.0682119013747098)) ;
#17862=DIRECTION('ref_axis',(0.703809019912964,0.707106781186548,0.0682119013747098)) ;
#17863=DIRECTION('center_axis',(0.,1.,0.)) ;
#17864=DIRECTION('ref_axis',(1.,0.,0.)) ;
#17865=DIRECTION('center_axis',(0.,1.,0.)) ;
#17866=DIRECTION('ref_axis',(1.,0.,0.)) ;
#17867=DIRECTION('center_axis',(-0.703809019912964,0.707106781186547,-0.0682119013747098)) ;
#17868=DIRECTION('ref_axis',(0.703809019912964,0.707106781186548,0.0682119013747098)) ;
#17869=DIRECTION('center_axis',(0.,-1.,0.)) ;
#17870=DIRECTION('ref_axis',(1.,0.,0.)) ;
#17871=DIRECTION('center_axis',(0.,1.,0.)) ;
#17872=DIRECTION('ref_axis',(1.,0.,0.)) ;
#17873=DIRECTION('center_axis',(0.995336261281429,0.,0.0964661960393706)) ;
#17874=DIRECTION('ref_axis',(0.0964661960393706,0.,-0.995336261281429)) ;
#17875=DIRECTION('',(-0.995336261281429,0.,-0.0964661960393706)) ;
#17876=DIRECTION('center_axis',(-0.999825160912746,0.,-0.0186988664309099)) ;
#17877=DIRECTION('ref_axis',(0.0186988664309099,0.,-0.999825160912746)) ;
#17878=DIRECTION('center_axis',(-0.995336261281429,0.,-0.0964661960393706)) ;
#17879=DIRECTION('ref_axis',(0.0964661960393706,0.,-0.995336261281429)) ;
#17880=DIRECTION('center_axis',(-0.999825160912746,0.,-0.0186988664309099)) ;
#17881=DIRECTION('ref_axis',(0.0186988664309099,0.,-0.999825160912746)) ;
#17882=DIRECTION('center_axis',(0.995336261281429,0.,0.0964661960393706)) ;
#17883=DIRECTION('ref_axis',(0.0964661960393706,0.,-0.995336261281429)) ;
#17884=DIRECTION('center_axis',(0.995336261281429,0.,0.0964661960393706)) ;
#17885=DIRECTION('ref_axis',(0.0964661960393706,0.,-0.995336261281429)) ;
#17886=DIRECTION('center_axis',(0.995336261281429,0.,0.0964661960393706)) ;
#17887=DIRECTION('ref_axis',(0.0964661960393706,0.,-0.995336261281429)) ;
#17888=DIRECTION('center_axis',(0.998247213677188,0.,-0.0591819261745526)) ;
#17889=DIRECTION('ref_axis',(0.0591819261745526,0.,0.998247213677188)) ;
#17890=DIRECTION('center_axis',(0.998247213677188,0.,-0.0591819261745526)) ;
#17891=DIRECTION('ref_axis',(0.0591819261745526,0.,0.998247213677188)) ;
#17892=DIRECTION('',(-0.998247213677188,0.,0.0591819261745526)) ;
#17893=DIRECTION('center_axis',(-0.990611994413054,0.,0.136703608310067)) ;
#17894=DIRECTION('ref_axis',(0.136703608310067,0.,0.990611994413054)) ;
#17895=DIRECTION('center_axis',(0.998247213677188,0.,-0.0591819261745526)) ;
#17896=DIRECTION('ref_axis',(0.0591819261745526,0.,0.998247213677188)) ;
#17897=DIRECTION('center_axis',(0.976965832926672,0.,-0.213395785557951)) ;
#17898=DIRECTION('ref_axis',(0.213395785557951,0.,0.976965832926672)) ;
#17899=DIRECTION('',(-0.976965832926672,0.,0.213395785557951)) ;
#17900=DIRECTION('center_axis',(-0.957391532867416,0.,0.288793096859637)) ;
#17901=DIRECTION('ref_axis',(0.288793096859637,0.,0.957391532867416)) ;
#17902=DIRECTION('center_axis',(0.932007869282798,0.,-0.362438038283702)) ;
#17903=DIRECTION('ref_axis',(0.362438038283702,0.,0.932007869282798)) ;
#17904=DIRECTION('',(-0.932007869282798,0.,0.362438038283702)) ;
#17905=DIRECTION('center_axis',(-0.932007869282798,0.,0.362438038283702)) ;
#17906=DIRECTION('ref_axis',(0.362438038283702,0.,0.932007869282798)) ;
#17907=DIRECTION('center_axis',(-0.900968867902422,0.,0.433883739117552)) ;
#17908=DIRECTION('ref_axis',(0.433883739117552,0.,0.900968867902422)) ;
#17909=DIRECTION('center_axis',(-0.932007869282798,0.,0.362438038283702)) ;
#17910=DIRECTION('ref_axis',(0.362438038283702,0.,0.932007869282798)) ;
#17911=DIRECTION('center_axis',(0.864462870524064,0.,-0.502696673437666)) ;
#17912=DIRECTION('ref_axis',(0.502696673437666,0.,0.864462870524064)) ;
#17913=DIRECTION('center_axis',(0.864462870524064,0.,-0.502696673437666)) ;
#17914=DIRECTION('ref_axis',(0.502696673437666,0.,0.864462870524064)) ;
#17915=DIRECTION('',(-0.864462870524064,0.,0.502696673437666)) ;
#17916=DIRECTION('center_axis',(-0.864462870524064,0.,0.502696673437666)) ;
#17917=DIRECTION('ref_axis',(0.502696673437666,0.,0.864462870524064)) ;
#17918=DIRECTION('center_axis',(-0.822711392173034,0.,0.568459290704891)) ;
#17919=DIRECTION('ref_axis',(0.568459290704891,0.,0.822711392173034)) ;
#17920=DIRECTION('center_axis',(-0.864462870524064,0.,0.502696673437666)) ;
#17921=DIRECTION('ref_axis',(0.502696673437666,0.,0.864462870524064)) ;
#17922=DIRECTION('center_axis',(0.864462870524064,0.,-0.502696673437666)) ;
#17923=DIRECTION('ref_axis',(0.502696673437666,0.,0.864462870524064)) ;
#17924=DIRECTION('center_axis',(0.775967776969404,0.,-0.630772549422659)) ;
#17925=DIRECTION('ref_axis',(0.630772549422659,0.,0.775967776969404)) ;
#17926=DIRECTION('center_axis',(0.775967776969404,0.,-0.630772549422659)) ;
#17927=DIRECTION('ref_axis',(0.630772549422659,0.,0.775967776969404)) ;
#17928=DIRECTION('',(-0.775967776969404,0.,0.630772549422659)) ;
#17929=DIRECTION('center_axis',(-0.724515660859275,0.,0.689258338483945)) ;
#17930=DIRECTION('ref_axis',(0.689258338483945,0.,0.724515660859275)) ;
#17931=DIRECTION('center_axis',(0.775967776969404,0.,-0.630772549422659)) ;
#17932=DIRECTION('ref_axis',(0.630772549422659,0.,0.775967776969404)) ;
#17933=DIRECTION('center_axis',(0.668667250537987,0.,-0.743561771514626)) ;
#17934=DIRECTION('ref_axis',(0.743561771514626,0.,0.668667250537987)) ;
#17935=DIRECTION('',(-0.668667250537987,0.,0.743561771514626)) ;
#17936=DIRECTION('center_axis',(-0.608761429008721,0.,0.793353340291235)) ;
#17937=DIRECTION('ref_axis',(0.793353340291235,0.,0.608761429008721)) ;
#17938=DIRECTION('center_axis',(0.545161699271658,0.,-0.838330914166499)) ;
#17939=DIRECTION('ref_axis',(0.838330914166499,0.,0.545161699271658)) ;
#17940=DIRECTION('',(-0.545161699271658,0.,0.838330914166499)) ;
#17941=DIRECTION('center_axis',(-0.545161699271658,0.,0.838330914166499)) ;
#17942=DIRECTION('ref_axis',(0.838330914166499,0.,0.545161699271658)) ;
#17943=DIRECTION('center_axis',(-0.478253978621312,0.,0.878221573370232)) ;
#17944=DIRECTION('ref_axis',(0.878221573370232,0.,0.478253978621312)) ;
#17945=DIRECTION('center_axis',(-0.545161699271658,0.,0.838330914166499)) ;
#17946=DIRECTION('ref_axis',(0.838330914166499,0.,0.545161699271658)) ;
#17947=DIRECTION('center_axis',(0.408444256935997,0.,-0.912783265061319)) ;
#17948=DIRECTION('ref_axis',(0.912783265061319,0.,0.408444256935996)) ;
#17949=DIRECTION('center_axis',(0.408444256935997,0.,-0.912783265061319)) ;
#17950=DIRECTION('ref_axis',(0.912783265061319,0.,0.408444256935996)) ;
#17951=DIRECTION('',(-0.408444256935996,0.,0.912783265061319)) ;
#17952=DIRECTION('center_axis',(-0.408444256935997,0.,0.912783265061319)) ;
#17953=DIRECTION('ref_axis',(0.912783265061319,0.,0.408444256935996)) ;
#17954=DIRECTION('center_axis',(-0.336156133168625,0.,0.941806272082066)) ;
#17955=DIRECTION('ref_axis',(0.941806272082065,0.,0.336156133168625)) ;
#17956=DIRECTION('center_axis',(-0.408444256935997,0.,0.912783265061319)) ;
#17957=DIRECTION('ref_axis',(0.912783265061319,0.,0.408444256935996)) ;
#17958=DIRECTION('center_axis',(0.408444256935997,0.,-0.912783265061319)) ;
#17959=DIRECTION('ref_axis',(0.912783265061319,0.,0.408444256935996)) ;
#17960=DIRECTION('center_axis',(0.261828244987421,0.,-0.965114485502527)) ;
#17961=DIRECTION('ref_axis',(0.965114485502527,0.,0.261828244987421)) ;
#17962=DIRECTION('center_axis',(0.261828244987421,0.,-0.965114485502527)) ;
#17963=DIRECTION('ref_axis',(0.965114485502527,0.,0.261828244987421)) ;
#17964=DIRECTION('',(-0.261828244987421,0.,0.965114485502527)) ;
#17965=DIRECTION('center_axis',(-0.185911607162916,0.,0.982566473233288)) ;
#17966=DIRECTION('ref_axis',(0.982566473233288,0.,0.185911607162916)) ;
#17967=DIRECTION('center_axis',(0.261828244987421,0.,-0.965114485502527)) ;
#17968=DIRECTION('ref_axis',(0.965114485502527,0.,0.261828244987421)) ;
#17969=DIRECTION('center_axis',(0.108866874851964,0.,-0.99405633822232)) ;
#17970=DIRECTION('ref_axis',(0.99405633822232,0.,0.108866874851965)) ;
#17971=DIRECTION('',(-0.108866874851965,0.,0.99405633822232)) ;
#17972=DIRECTION('center_axis',(-0.0311615483847374,0.,0.999514361028528)) ;
#17973=DIRECTION('ref_axis',(0.999514361028528,0.,0.0311615483847374)) ;
#17974=DIRECTION('center_axis',(-0.0467328634842026,0.,-0.998907422872894)) ;
#17975=DIRECTION('ref_axis',(0.998907422872894,0.,-0.0467328634842026)) ;
#17976=DIRECTION('',(0.0467328634842026,0.,0.998907422872894)) ;
#17977=DIRECTION('center_axis',(0.0467328634842026,0.,0.998907422872894)) ;
#17978=DIRECTION('ref_axis',(0.998907422872894,0.,-0.0467328634842026)) ;
#17979=DIRECTION('center_axis',(0.124343704647499,0.,0.99223920660017)) ;
#17980=DIRECTION('ref_axis',(0.99223920660017,0.,-0.124343704647499)) ;
#17981=DIRECTION('center_axis',(0.0467328634842026,0.,0.998907422872894)) ;
#17982=DIRECTION('ref_axis',(0.998907422872894,0.,-0.0467328634842026)) ;
#17983=DIRECTION('center_axis',(-0.201200039678648,0.,-0.979550174331724)) ;
#17984=DIRECTION('ref_axis',(0.979550174331724,0.,-0.201200039678648)) ;
#17985=DIRECTION('center_axis',(-0.201200039678648,0.,-0.979550174331724)) ;
#17986=DIRECTION('ref_axis',(0.979550174331724,0.,-0.201200039678648)) ;
#17987=DIRECTION('',(0.201200039678648,0.,0.979550174331724)) ;
#17988=DIRECTION('center_axis',(0.201200039678648,0.,0.979550174331724)) ;
#17989=DIRECTION('ref_axis',(0.979550174331724,0.,-0.201200039678648)) ;
#17990=DIRECTION('center_axis',(0.276835511424842,0.,0.960917321945102)) ;
#17991=DIRECTION('ref_axis',(0.960917321945102,0.,-0.276835511424842)) ;
#17992=DIRECTION('center_axis',(0.201200039678648,0.,0.979550174331724)) ;
#17993=DIRECTION('ref_axis',(0.979550174331724,0.,-0.201200039678648)) ;
#17994=DIRECTION('center_axis',(-0.201200039678648,0.,-0.979550174331724)) ;
#17995=DIRECTION('ref_axis',(0.979550174331724,0.,-0.201200039678648)) ;
#17996=DIRECTION('center_axis',(-0.350791170819065,0.,-0.936453711870154)) ;
#17997=DIRECTION('ref_axis',(0.936453711870154,0.,-0.350791170819065)) ;
#17998=DIRECTION('center_axis',(-0.350791170819065,0.,-0.936453711870154)) ;
#17999=DIRECTION('ref_axis',(0.936453711870154,0.,-0.350791170819065)) ;
#18000=DIRECTION('',(0.350791170819065,0.,0.936453711870154)) ;
#18001=DIRECTION('center_axis',(0.248046815666529,-0.707106781186547,0.6621727699307)) ;
#18002=DIRECTION('ref_axis',(-0.248046815666529,-0.707106781186548,-0.662172769930699)) ;
#18003=DIRECTION('center_axis',(0.248046815666529,-0.707106781186547,0.6621727699307)) ;
#18004=DIRECTION('ref_axis',(-0.248046815666529,-0.707106781186548,-0.662172769930699)) ;
#18005=DIRECTION('center_axis',(-0.350791170819065,0.,-0.936453711870154)) ;
#18006=DIRECTION('ref_axis',(0.936453711870154,0.,-0.350791170819065)) ;
#18007=DIRECTION('center_axis',(-0.350791170819065,0.,-0.936453711870154)) ;
#18008=DIRECTION('ref_axis',(0.936453711870154,0.,-0.350791170819065)) ;
#18009=DIRECTION('center_axis',(0.,1.,0.)) ;
#18010=DIRECTION('ref_axis',(1.,0.,0.)) ;
#18011=DIRECTION('',(0.,-1.,0.)) ;
#18012=DIRECTION('center_axis',(0.,-1.,0.)) ;
#18013=DIRECTION('ref_axis',(1.,0.,0.)) ;
#18014=DIRECTION('center_axis',(0.,-1.,0.)) ;
#18015=DIRECTION('ref_axis',(-1.,0.,0.)) ;
#18016=DIRECTION('center_axis',(0.,0.,1.)) ;
#18017=DIRECTION('ref_axis',(-1.,0.,0.)) ;
#18018=DIRECTION('center_axis',(0.,0.,1.)) ;
#18019=DIRECTION('ref_axis',(-1.,0.,0.)) ;
#18020=DIRECTION('center_axis',(0.,0.,1.)) ;
#18021=DIRECTION('ref_axis',(-1.,0.,0.)) ;
#18022=DIRECTION('center_axis',(0.,0.,1.)) ;
#18023=DIRECTION('ref_axis',(-1.,0.,0.)) ;
#18024=DIRECTION('center_axis',(0.,0.,1.)) ;
#18025=DIRECTION('ref_axis',(-1.,0.,0.)) ;
#18026=DIRECTION('center_axis',(0.,0.,1.)) ;
#18027=DIRECTION('ref_axis',(-1.,0.,0.)) ;
#18028=DIRECTION('center_axis',(5.94762334620619E-17,0.,1.)) ;
#18029=DIRECTION('ref_axis',(1.,0.,0.)) ;
#18030=DIRECTION('center_axis',(0.,-1.,0.)) ;
#18031=DIRECTION('ref_axis',(-1.,0.,0.)) ;
#18032=DIRECTION('center_axis',(0.,-1.,0.)) ;
#18033=DIRECTION('ref_axis',(1.,0.,0.)) ;
#18034=DIRECTION('center_axis',(0.,1.,0.)) ;
#18035=DIRECTION('ref_axis',(1.,0.,0.)) ;
#18036=DIRECTION('',(0.,-1.,0.)) ;
#18037=DIRECTION('center_axis',(0.577350269189626,0.577350269189626,0.577350269189626)) ;
#18038=DIRECTION('ref_axis',(-0.707106781186548,0.,0.707106781186547)) ;
#18039=DIRECTION('center_axis',(-0.408248290463863,0.816496580927726,-0.408248290463863)) ;
#18040=DIRECTION('ref_axis',(0.707106781186548,0.,-0.707106781186547)) ;
#18041=DIRECTION('center_axis',(0.,0.,1.)) ;
#18042=DIRECTION('ref_axis',(1.,0.,0.)) ;
#18043=DIRECTION('center_axis',(0.,0.,1.)) ;
#18044=DIRECTION('ref_axis',(-0.999995485023846,-0.00300498451297073,0.)) ;
#18045=DIRECTION('center_axis',(-0.976965832926672,0.,0.213395785557951)) ;
#18046=DIRECTION('ref_axis',(-0.213395785557951,0.,-0.976965832926672)) ;
#18047=DIRECTION('center_axis',(0.,0.,1.)) ;
#18048=DIRECTION('ref_axis',(1.,0.,0.)) ;
#18049=DIRECTION('center_axis',(0.,0.,1.)) ;
#18050=DIRECTION('ref_axis',(-0.999998402547297,-0.00178742911851967,0.)) ;
#18051=DIRECTION('center_axis',(-0.864462870524064,0.,0.502696673437666)) ;
#18052=DIRECTION('ref_axis',(0.,1.,0.)) ;
#18053=DIRECTION('center_axis',(0.,0.,1.)) ;
#18054=DIRECTION('ref_axis',(1.,0.,0.)) ;
#18055=DIRECTION('center_axis',(0.,0.,1.)) ;
#18056=DIRECTION('ref_axis',(1.,0.,0.)) ;
#18057=DIRECTION('center_axis',(-0.668667250537987,0.,0.743561771514626)) ;
#18058=DIRECTION('ref_axis',(0.,1.,0.)) ;
#18059=DIRECTION('center_axis',(0.,1.,0.)) ;
#18060=DIRECTION('ref_axis',(-1.,0.,0.)) ;
#18061=DIRECTION('center_axis',(0.,0.,1.)) ;
#18062=DIRECTION('ref_axis',(1.,0.,0.)) ;
#18063=DIRECTION('center_axis',(0.,1.,0.)) ;
#18064=DIRECTION('ref_axis',(-1.,0.,0.)) ;
#18065=DIRECTION('center_axis',(0.,0.,1.)) ;
#18066=DIRECTION('ref_axis',(1.,0.,0.)) ;
#18067=DIRECTION('center_axis',(-0.408444256935997,0.,0.912783265061319)) ;
#18068=DIRECTION('ref_axis',(0.,1.,0.)) ;
#18069=DIRECTION('center_axis',(0.,1.,0.)) ;
#18070=DIRECTION('ref_axis',(-1.,0.,0.)) ;
#18071=DIRECTION('center_axis',(0.,0.,1.)) ;
#18072=DIRECTION('ref_axis',(1.,0.,0.)) ;
#18073=DIRECTION('center_axis',(0.,1.,0.)) ;
#18074=DIRECTION('ref_axis',(-1.,0.,0.)) ;
#18075=DIRECTION('center_axis',(0.,0.,1.)) ;
#18076=DIRECTION('ref_axis',(1.,0.,0.)) ;
#18077=DIRECTION('center_axis',(-0.108866874851964,0.,0.99405633822232)) ;
#18078=DIRECTION('ref_axis',(0.,1.,0.)) ;
#18079=DIRECTION('center_axis',(0.,1.,0.)) ;
#18080=DIRECTION('ref_axis',(-1.,0.,0.)) ;
#18081=DIRECTION('center_axis',(0.,0.,1.)) ;
#18082=DIRECTION('ref_axis',(1.,0.,0.)) ;
#18083=DIRECTION('center_axis',(0.,1.,0.)) ;
#18084=DIRECTION('ref_axis',(-1.,0.,0.)) ;
#18085=DIRECTION('center_axis',(0.,0.,1.)) ;
#18086=DIRECTION('ref_axis',(1.,0.,0.)) ;
#18087=DIRECTION('center_axis',(0.201200039678648,0.,0.979550174331724)) ;
#18088=DIRECTION('ref_axis',(0.,1.,0.)) ;
#18089=DIRECTION('center_axis',(0.,1.,0.)) ;
#18090=DIRECTION('ref_axis',(-1.,0.,0.)) ;
#18091=DIRECTION('center_axis',(0.,0.,1.)) ;
#18092=DIRECTION('ref_axis',(1.,0.,0.)) ;
#18093=DIRECTION('center_axis',(0.,1.,0.)) ;
#18094=DIRECTION('ref_axis',(-1.,0.,0.)) ;
#21616=CARTESIAN_POINT('',(0.,0.,0.)) ;
#21617=CARTESIAN_POINT('Origin',(-8.33803164073718,5.6,3.88808800801444)) ;
#21618=CARTESIAN_POINT('',(-9.43554118180326,5.6,3.81410958366699)) ;
#21619=CARTESIAN_POINT('Origin',(-8.49738695853213,5.6,3.46268140924831)) ;
#21620=CARTESIAN_POINT('',(-8.33803164073718,5.6,4.98808800801443)) ;
#21621=CARTESIAN_POINT('Origin',(-8.33803164073718,5.6,3.88808800801444)) ;
#21622=CARTESIAN_POINT('Origin',(-8.84043936189492,5.6,2.54688670510862)) ;
#21623=CARTESIAN_POINT('',(-8.84043936189492,5.6,3.94688670510862)) ;
#21624=CARTESIAN_POINT('Origin',(-8.84043936189492,5.6,2.54688670510862)) ;
#21625=CARTESIAN_POINT('Origin',(-8.33803164073718,5.6,3.88808800801444)) ;
#21626=CARTESIAN_POINT('',(-9.37115550181876,5.6,3.51039092348254)) ;
#21627=CARTESIAN_POINT('Origin',(-8.58923550131605,5.6,3.21748735656153)) ;
#21628=CARTESIAN_POINT('',(-8.33803164073718,5.6,2.78808800801444)) ;
#21629=CARTESIAN_POINT('Origin',(-8.33803164073718,5.6,3.88808800801444)) ;
#21630=CARTESIAN_POINT('Origin',(-8.84043936189492,5.6,2.54688670510862)) ;
#21631=CARTESIAN_POINT('',(-8.84043936189492,5.6,3.64688670510861)) ;
#21632=CARTESIAN_POINT('Origin',(-8.84043936189492,5.6,2.54688670510862)) ;
#21633=CARTESIAN_POINT('Origin',(-8.84043936189492,5.6,2.54688670510862)) ;
#21634=CARTESIAN_POINT('',(-8.20946536255214,4.73397459621556,2.79562715648993)) ;
#21635=CARTESIAN_POINT('',(-9.1527027256478,4.73397459621556,3.14895945125955)) ;
#21636=CARTESIAN_POINT('Origin',(-8.68108404409997,5.6,2.97229330387474)) ;
#21637=CARTESIAN_POINT('Ctrl Pts',(-9.1527027256478,4.73397459621556,3.14895945125955)) ;
#21638=CARTESIAN_POINT('Ctrl Pts',(-9.13645723854168,4.71566855398674,3.13105359647328)) ;
#21639=CARTESIAN_POINT('Ctrl Pts',(-9.1190870121684,4.69851255867057,3.11309468626371)) ;
#21640=CARTESIAN_POINT('Ctrl Pts',(-9.05446121186005,4.64303800908893,3.05094049520305)) ;
#21641=CARTESIAN_POINT('Ctrl Pts',(-8.99680270458556,4.6083948945016,3.00378876637968)) ;
#21642=CARTESIAN_POINT('Ctrl Pts',(-8.86677648250724,4.56256392827545,2.92041371476685)) ;
#21643=CARTESIAN_POINT('Ctrl Pts',(-8.79430324329648,4.55136544237033,2.88436092742056)) ;
#21644=CARTESIAN_POINT('Ctrl Pts',(-8.65350061397982,4.55136544237033,2.83161692249397)) ;
#21645=CARTESIAN_POINT('Ctrl Pts',(-8.57517702407941,4.56256392827545,2.81118192451869)) ;
#21646=CARTESIAN_POINT('Ctrl Pts',(-8.42237405343921,4.6083948945016,2.78861048630727)) ;
#21647=CARTESIAN_POINT('Ctrl Pts',(-8.34792716046905,4.64303800908893,2.78627615144598)) ;
#21648=CARTESIAN_POINT('Ctrl Pts',(-8.25837107871867,4.69851255867057,2.79067453221843)) ;
#21649=CARTESIAN_POINT('Ctrl Pts',(-8.23347682647838,4.71566855398674,2.79280136685503)) ;
#21650=CARTESIAN_POINT('Ctrl Pts',(-8.20946536255214,4.73397459621556,2.79562715648993)) ;
#21651=CARTESIAN_POINT('Origin',(-8.33803164073718,4.7,3.88808800801444)) ;
#21652=CARTESIAN_POINT('Origin',(-8.33803164073718,4.73397459621556,3.88808800801444)) ;
#21653=CARTESIAN_POINT('Origin',(-8.33803164073718,5.6,3.88808800801444)) ;
#21654=CARTESIAN_POINT('Origin',(-9.12860070072158,5.6,1.14396208275687)) ;
#21655=CARTESIAN_POINT('',(-9.91316825898094,5.6,2.30346790271938)) ;
#21656=CARTESIAN_POINT('Origin',(-8.93183931414709,5.6,2.10190250279173)) ;
#21657=CARTESIAN_POINT('',(-9.12860070072158,5.6,2.54396208275687)) ;
#21658=CARTESIAN_POINT('Origin',(-9.12860070072158,5.6,1.14396208275687)) ;
#21659=CARTESIAN_POINT('Origin',(-8.84043936189492,5.6,2.54688670510862)) ;
#21660=CARTESIAN_POINT('',(-9.6192382673711,5.6,3.32372147829343)) ;
#21661=CARTESIAN_POINT('Origin',(-8.84043936189492,5.6,2.54688670510862)) ;
#21662=CARTESIAN_POINT('',(-7.74292982082884,5.6,2.62086512945606)) ;
#21663=CARTESIAN_POINT('Ctrl Pts',(-7.74292982082884,5.6,2.62086512945606)) ;
#21664=CARTESIAN_POINT('Ctrl Pts',(-7.74292982082884,5.47323659419775,2.62086512945606)) ;
#21665=CARTESIAN_POINT('Ctrl Pts',(-7.76540878473659,5.33803946527454,2.60956776356783)) ;
#21666=CARTESIAN_POINT('Ctrl Pts',(-7.85827962884553,5.08718469591568,2.57190072801271)) ;
#21667=CARTESIAN_POINT('Ctrl Pts',(-7.92885376828481,4.97144567551952,2.54652928381717)) ;
#21668=CARTESIAN_POINT('Ctrl Pts',(-8.04906993302529,4.83434481308716,2.5176859704715)) ;
#21669=CARTESIAN_POINT('Ctrl Pts',(-8.09402492641871,4.79043643796436,2.50863906272968)) ;
#21670=CARTESIAN_POINT('Ctrl Pts',(-8.19142307953697,4.711142531426,2.49491730637113)) ;
#21671=CARTESIAN_POINT('Ctrl Pts',(-8.24386922105279,4.67574116355534,2.49035537389413)) ;
#21672=CARTESIAN_POINT('Ctrl Pts',(-8.37274894896879,4.60209590056535,2.48630683631571)) ;
#21673=CARTESIAN_POINT('Ctrl Pts',(-8.46381978450228,4.56343058934306,2.49058271315158)) ;
#21674=CARTESIAN_POINT('Ctrl Pts',(-8.64959407180091,4.51264465486516,2.519960558875)) ;
#21675=CARTESIAN_POINT('Ctrl Pts',(-8.7442527880297,4.50047177654324,2.54525472945496)) ;
#21676=CARTESIAN_POINT('Ctrl Pts',(-8.91402577173804,4.50047177654324,2.60885089333748)) ;
#21677=CARTESIAN_POINT('Ctrl Pts',(-9.00200639087887,4.51264465486516,2.65197256166106)) ;
#21678=CARTESIAN_POINT('Ctrl Pts',(-9.16136120100629,4.56343058934306,2.75187845803316)) ;
#21679=CARTESIAN_POINT('Ctrl Pts',(-9.23282794266408,4.60209590056535,2.80848839571465)) ;
#21680=CARTESIAN_POINT('Ctrl Pts',(-9.32732933695259,4.67574116355534,2.89621445456693)) ;
#21681=CARTESIAN_POINT('Ctrl Pts',(-9.36387082989461,4.711142531426,2.93411073778033)) ;
#21682=CARTESIAN_POINT('Ctrl Pts',(-9.42828324602872,4.79043643796436,3.00844597489019)) ;
#21683=CARTESIAN_POINT('Ctrl Pts',(-9.4562306030012,4.83434481308716,3.0448017613477)) ;
#21684=CARTESIAN_POINT('Ctrl Pts',(-9.52791046153494,4.97144567551952,3.14552842549503)) ;
#21685=CARTESIAN_POINT('Ctrl Pts',(-9.56444665447068,5.08718469591569,3.2110228981162)) ;
#21686=CARTESIAN_POINT('Ctrl Pts',(-9.6097139388173,5.33803946527454,3.30043582906525)) ;
#21687=CARTESIAN_POINT('Ctrl Pts',(-9.6192382673711,5.47323659419775,3.32372147829343)) ;
#21688=CARTESIAN_POINT('Ctrl Pts',(-9.6192382673711,5.6,3.32372147829343)) ;
#21689=CARTESIAN_POINT('Origin',(-8.68108404409997,5.6,2.97229330387474)) ;
#21690=CARTESIAN_POINT('Origin',(-8.33803164073718,5.6,3.88808800801444)) ;
#21691=CARTESIAN_POINT('Origin',(-8.33803164073718,5.6,3.88808800801444)) ;
#21692=CARTESIAN_POINT('Origin',(-8.33803164073718,4.7,3.88808800801444)) ;
#21693=CARTESIAN_POINT('Origin',(-9.12860070072158,5.6,1.14396208275687)) ;
#21694=CARTESIAN_POINT('',(-10.1505515711168,5.6,0.737002111139838)) ;
#21695=CARTESIAN_POINT('Origin',(-9.14983022680858,5.6,0.690184385194045)) ;
#21696=CARTESIAN_POINT('',(-10.0185296933033,5.6,1.7905116850014)) ;
#21697=CARTESIAN_POINT('Origin',(-9.12860070072158,5.6,1.14396208275687)) ;
#21698=CARTESIAN_POINT('Origin',(-9.03720074846941,5.6,1.58894628507375)) ;
#21699=CARTESIAN_POINT('Origin',(-8.84043936189492,5.6,2.54688670510862)) ;
#21700=CARTESIAN_POINT('',(-8.84043936189492,5.6,1.14688670510861)) ;
#21701=CARTESIAN_POINT('Origin',(-8.84043936189492,5.6,2.54688670510862)) ;
#21702=CARTESIAN_POINT('Origin',(-9.19553212146245,5.6,-0.286686245139542)) ;
#21703=CARTESIAN_POINT('',(-9.19553212146245,5.6,1.11331375486046)) ;
#21704=CARTESIAN_POINT('Origin',(-9.19553212146245,5.6,-0.286686245139542)) ;
#21705=CARTESIAN_POINT('Origin',(-9.12860070072158,5.6,1.14396208275687)) ;
#21706=CARTESIAN_POINT('',(-9.99613400321582,5.6,0.467658919180464)) ;
#21707=CARTESIAN_POINT('Origin',(-9.16206641109202,5.6,0.428637918808661)) ;
#21708=CARTESIAN_POINT('',(-9.12860070072158,5.6,0.0439620827568656)) ;
#21709=CARTESIAN_POINT('Origin',(-9.12860070072158,5.6,1.14396208275687)) ;
#21710=CARTESIAN_POINT('Origin',(-9.19553212146245,5.6,-0.286686245139542)) ;
#21711=CARTESIAN_POINT('',(-9.19553212146245,5.6,0.813313754860457)) ;
#21712=CARTESIAN_POINT('Origin',(-9.19553212146245,5.6,-0.286686245139542)) ;
#21713=CARTESIAN_POINT('Origin',(-9.03961155374625,5.6,-1.71038678589882)) ;
#21714=CARTESIAN_POINT('',(-10.1419381783659,5.6,-0.847324787746512)) ;
#21715=CARTESIAN_POINT('Origin',(-9.14607672781936,5.6,-0.738260220942957)) ;
#21716=CARTESIAN_POINT('',(-9.03961155374625,5.6,-0.310386785898815)) ;
#21717=CARTESIAN_POINT('Origin',(-9.03961155374625,5.6,-1.71038678589882)) ;
#21718=CARTESIAN_POINT('Origin',(-9.19553212146245,5.6,-0.286686245139542)) ;
#21719=CARTESIAN_POINT('',(-10.1750239396836,5.6,0.213909178369071)) ;
#21720=CARTESIAN_POINT('Origin',(-9.19553212146245,5.6,-0.286686245139542)) ;
#21721=CARTESIAN_POINT('Origin',(-9.17430259537545,5.6,0.167091452423278)) ;
#21722=CARTESIAN_POINT('Origin',(-9.12860070072158,5.6,1.14396208275687)) ;
#21723=CARTESIAN_POINT('',(-9.12860070072158,5.6,-0.256037917243135)) ;
#21724=CARTESIAN_POINT('Origin',(-9.12860070072158,5.6,1.14396208275687)) ;
#21725=CARTESIAN_POINT('Origin',(-9.03961155374625,5.6,-1.71038678589882)) ;
#21726=CARTESIAN_POINT('',(-9.88753682467885,5.6,-2.41111693004411)) ;
#21727=CARTESIAN_POINT('Origin',(-8.92066978252025,5.6,-2.14881322971911)) ;
#21728=CARTESIAN_POINT('',(-10.0849283979359,5.6,-1.36787737689896)) ;
#21729=CARTESIAN_POINT('Origin',(-9.03961155374625,5.6,-1.71038678589882)) ;
#21730=CARTESIAN_POINT('Origin',(-9.08906694738934,5.6,-1.2588128100954)) ;
#21731=CARTESIAN_POINT('Origin',(-9.19553212146245,5.6,-0.286686245139542)) ;
#21732=CARTESIAN_POINT('',(-9.19553212146245,5.6,-1.68668624513954)) ;
#21733=CARTESIAN_POINT('Origin',(-9.19553212146245,5.6,-0.286686245139542)) ;
#21734=CARTESIAN_POINT('Origin',(-8.66461770315499,5.6,-3.0926364251514)) ;
#21735=CARTESIAN_POINT('',(-8.66461770315499,5.6,-1.6926364251514)) ;
#21736=CARTESIAN_POINT('Origin',(-8.66461770315499,5.6,-3.0926364251514)) ;
#21737=CARTESIAN_POINT('Origin',(-9.03961155374625,5.6,-1.71038678589882)) ;
#21738=CARTESIAN_POINT('',(-9.65796579805327,5.6,-2.62013292001948)) ;
#21739=CARTESIAN_POINT('Origin',(-8.85211462845062,5.6,-2.40151160552511)) ;
#21740=CARTESIAN_POINT('',(-9.03961155374625,5.6,-2.81038678589882)) ;
#21741=CARTESIAN_POINT('Origin',(-9.03961155374625,5.6,-1.71038678589882)) ;
#21742=CARTESIAN_POINT('Origin',(-8.66461770315499,5.6,-3.0926364251514)) ;
#21743=CARTESIAN_POINT('',(-8.66461770315499,5.6,-1.9926364251514)) ;
#21744=CARTESIAN_POINT('Origin',(-8.66461770315499,5.6,-3.0926364251514)) ;
#21745=CARTESIAN_POINT('Origin',(-8.0796384750061,5.6,-4.39993660331612)) ;
#21746=CARTESIAN_POINT('',(-9.3935128789311,5.6,-3.91647610781443)) ;
#21747=CARTESIAN_POINT('Origin',(-8.47907208576222,5.6,-3.5072901547254)) ;
#21748=CARTESIAN_POINT('',(-8.0796384750061,5.6,-2.99993660331612)) ;
#21749=CARTESIAN_POINT('Origin',(-8.0796384750061,5.6,-4.39993660331612)) ;
#21750=CARTESIAN_POINT('Origin',(-8.66461770315499,5.6,-3.0926364251514)) ;
#21751=CARTESIAN_POINT('',(-9.75042651653959,5.6,-2.9165136816561)) ;
#21752=CARTESIAN_POINT('Origin',(-8.66461770315499,5.6,-3.0926364251514)) ;
#21753=CARTESIAN_POINT('Origin',(-8.78355947438099,5.6,-2.65420998133111)) ;
#21754=CARTESIAN_POINT('Origin',(-9.03961155374625,5.6,-1.71038678589882)) ;
#21755=CARTESIAN_POINT('',(-9.03961155374625,5.6,-3.11038678589882)) ;
#21756=CARTESIAN_POINT('Origin',(-9.03961155374625,5.6,-1.71038678589882)) ;
#21757=CARTESIAN_POINT('Origin',(-8.0796384750061,5.6,-4.39993660331612)) ;
#21758=CARTESIAN_POINT('',(-8.67183891837006,5.6,-5.32692022500506)) ;
#21759=CARTESIAN_POINT('Origin',(-7.83198567452591,5.6,-4.78076856363145)) ;
#21760=CARTESIAN_POINT('',(-9.17962488556776,5.6,-4.39446882683115)) ;
#21761=CARTESIAN_POINT('Origin',(-8.0796384750061,5.6,-4.39993660331612)) ;
#21762=CARTESIAN_POINT('Origin',(-8.26518409239888,5.6,-3.98528287374212)) ;
#21763=CARTESIAN_POINT('Origin',(-8.66461770315499,5.6,-3.0926364251514)) ;
#21764=CARTESIAN_POINT('',(-8.66461770315499,5.6,-4.4926364251514)) ;
#21765=CARTESIAN_POINT('Origin',(-8.66461770315499,5.6,-3.0926364251514)) ;
#21766=CARTESIAN_POINT('Origin',(-7.29885073067936,5.6,-5.60060514688023)) ;
#21767=CARTESIAN_POINT('',(-7.29885073067936,5.6,-4.20060514688023)) ;
#21768=CARTESIAN_POINT('Origin',(-7.29885073067936,5.6,-5.60060514688023)) ;
#21769=CARTESIAN_POINT('Origin',(-8.0796384750061,5.6,-4.39993660331612)) ;
#21770=CARTESIAN_POINT('',(-8.38923404227527,5.6,-5.45546992099363)) ;
#21771=CARTESIAN_POINT('Origin',(-7.68924460284273,5.6,-5.00027087509818)) ;
#21772=CARTESIAN_POINT('',(-8.0796384750061,5.6,-5.49993660331612)) ;
#21773=CARTESIAN_POINT('Origin',(-8.0796384750061,5.6,-4.39993660331612)) ;
#21774=CARTESIAN_POINT('Origin',(-7.29885073067936,5.6,-5.60060514688023)) ;
#21775=CARTESIAN_POINT('',(-7.29885073067936,5.6,-4.50060514688023)) ;
#21776=CARTESIAN_POINT('Origin',(-7.29885073067936,5.6,-5.60060514688023)) ;
#21777=CARTESIAN_POINT('Origin',(-6.34117671405231,5.6,-6.66554407990531)) ;
#21778=CARTESIAN_POINT('',(-7.7400045754612,5.6,-6.60826743417404)) ;
#21779=CARTESIAN_POINT('Origin',(-6.99509256607175,5.6,-5.9383859471302)) ;
#21780=CARTESIAN_POINT('',(-6.34117671405231,5.6,-5.26554407990531)) ;
#21781=CARTESIAN_POINT('Origin',(-6.34117671405231,5.6,-6.66554407990531)) ;
#21782=CARTESIAN_POINT('Origin',(-7.29885073067936,5.6,-5.60060514688023)) ;
#21783=CARTESIAN_POINT('',(-8.38635677500372,5.6,-5.76592484793852)) ;
#21784=CARTESIAN_POINT('Origin',(-7.29885073067936,5.6,-5.60060514688023)) ;
#21785=CARTESIAN_POINT('Origin',(-7.54650353115956,5.6,-5.21977318656491)) ;
#21786=CARTESIAN_POINT('Origin',(-8.0796384750061,5.6,-4.39993660331612)) ;
#21787=CARTESIAN_POINT('',(-8.0796384750061,5.6,-5.79993660331612)) ;
#21788=CARTESIAN_POINT('Origin',(-8.0796384750061,5.6,-4.39993660331612)) ;
#21789=CARTESIAN_POINT('Origin',(-6.34117671405231,5.6,-6.66554407990531)) ;
#21790=CARTESIAN_POINT('',(-6.62059267994042,5.6,-7.7294645271225)) ;
#21791=CARTESIAN_POINT('Origin',(-5.98867470720626,5.6,-6.95208766603628)) ;
#21792=CARTESIAN_POINT('',(-7.38984688804938,5.6,-6.99764476669919)) ;
#21793=CARTESIAN_POINT('Origin',(-6.34117671405231,5.6,-6.66554407990531)) ;
#21794=CARTESIAN_POINT('Origin',(-6.64493487865992,5.6,-6.32776327965534)) ;
#21795=CARTESIAN_POINT('Origin',(-7.29885073067936,5.6,-5.60060514688023)) ;
#21796=CARTESIAN_POINT('',(-7.29885073067936,5.6,-7.00060514688023)) ;
#21797=CARTESIAN_POINT('Origin',(-7.29885073067936,5.6,-5.60060514688023)) ;
#21798=CARTESIAN_POINT('Origin',(-5.22982547448501,5.6,-7.56894480799191)) ;
#21799=CARTESIAN_POINT('Origin',(-6.34117671405231,5.6,-6.66554407990531)) ;
#21800=CARTESIAN_POINT('',(-5.78550109426866,4.76502012796642,-7.11724444394861)) ;
#21801=CARTESIAN_POINT('Origin',(-5.78550109426866,5.6,-7.11724444394861)) ;
#21802=CARTESIAN_POINT('Origin',(-5.22982547448501,5.6,-7.56894480799191)) ;
#21803=CARTESIAN_POINT('Origin',(-3.99173039988154,5.6,-8.28891358470226)) ;
#21804=CARTESIAN_POINT('',(-5.34073196819012,5.6,-8.66333950354468)) ;
#21805=CARTESIAN_POINT('Origin',(-4.83712244512243,5.6,-7.79730685018094)) ;
#21806=CARTESIAN_POINT('Origin',(-5.22982547448501,5.6,-7.56894480799191)) ;
#21807=CARTESIAN_POINT('',(-6.21424545406522,5.6,-8.05977808294716)) ;
#21808=CARTESIAN_POINT('Origin',(-5.22982547448501,5.6,-7.56894480799191)) ;
#21809=CARTESIAN_POINT('Origin',(-5.58232748133106,5.6,-7.28240122186094)) ;
#21810=CARTESIAN_POINT('Origin',(-6.34117671405231,5.6,-6.66554407990531)) ;
#21811=CARTESIAN_POINT('Origin',(-3.99173039988154,5.6,-8.28891358470226)) ;
#21812=CARTESIAN_POINT('',(-4.88804295231181,5.6,-8.92658419587697)) ;
#21813=CARTESIAN_POINT('Origin',(-4.38443342924412,5.6,-8.06055154251323)) ;
#21814=CARTESIAN_POINT('',(-3.99173039988154,5.6,-9.38891358470226)) ;
#21815=CARTESIAN_POINT('Origin',(-3.99173039988154,5.6,-8.28891358470226)) ;
#21816=CARTESIAN_POINT('',(-3.93143962342431,5.6,-9.38726007933598)) ;
#21817=CARTESIAN_POINT('Origin',(-3.56834343193086,5.6,-8.453559771882)) ;
#21818=CARTESIAN_POINT('Origin',(-5.22982547448501,5.6,-7.56894480799191)) ;
#21819=CARTESIAN_POINT('Origin',(-2.6568964911086,5.6,-8.80800210238025)) ;
#21820=CARTESIAN_POINT('Origin',(-3.99173039988154,5.6,-8.28891358470226)) ;
#21821=CARTESIAN_POINT('',(-3.02168497866884,5.6,-7.77025003211321)) ;
#21822=CARTESIAN_POINT('Origin',(-3.32431344549507,5.6,-8.54845784354125)) ;
#21823=CARTESIAN_POINT('Origin',(-2.6568964911086,5.6,-8.80800210238025)) ;
#21824=CARTESIAN_POINT('Origin',(-1.25767319645268,5.6,-9.11363034860009)) ;
#21825=CARTESIAN_POINT('',(-2.42686958009725,5.6,-9.88368217573411)) ;
#21826=CARTESIAN_POINT('Origin',(-2.21308628796886,5.6,-8.90494226522496)) ;
#21827=CARTESIAN_POINT('Origin',(-2.6568964911086,5.6,-8.80800210238025)) ;
#21828=CARTESIAN_POINT('',(-3.44337965055272,5.6,-9.57705622265449)) ;
#21829=CARTESIAN_POINT('',(-2.71718726756582,5.6,-7.70965560774652)) ;
#21830=CARTESIAN_POINT('Origin',(-3.08028345905927,5.6,-8.64335591520051)) ;
#21831=CARTESIAN_POINT('',(-2.6568964911086,5.6,-9.90800210238025)) ;
#21832=CARTESIAN_POINT('Origin',(-2.6568964911086,5.6,-8.80800210238025)) ;
#21833=CARTESIAN_POINT('Origin',(-3.08028345905927,5.6,-8.64335591520051)) ;
#21834=CARTESIAN_POINT('',(-2.6568964911086,5.6,-7.70800210238025)) ;
#21835=CARTESIAN_POINT('Origin',(-2.6568964911086,5.6,-8.80800210238025)) ;
#21836=CARTESIAN_POINT('Origin',(-3.99173039988154,5.6,-8.28891358470226)) ;
#21837=CARTESIAN_POINT('Origin',(-1.25767319645268,5.6,-9.11363034860009)) ;
#21838=CARTESIAN_POINT('',(-1.9152666917208,5.6,-9.99543009626452)) ;
#21839=CARTESIAN_POINT('',(-1.48770010746402,5.6,-8.03795027524622)) ;
#21840=CARTESIAN_POINT('Origin',(-1.70148339959241,5.6,-9.01669018575537)) ;
#21841=CARTESIAN_POINT('',(-1.25767319645268,5.6,-10.2136303486001)) ;
#21842=CARTESIAN_POINT('Origin',(-1.25767319645268,5.6,-9.11363034860009)) ;
#21843=CARTESIAN_POINT('Origin',(-1.70148339959241,5.6,-9.01669018575537)) ;
#21844=CARTESIAN_POINT('',(-1.25767319645268,5.6,-8.01363034860009)) ;
#21845=CARTESIAN_POINT('Origin',(-1.25767319645268,5.6,-9.11363034860009)) ;
#21846=CARTESIAN_POINT('',(-0.863484809736792,5.6,-10.1405750967625)) ;
#21847=CARTESIAN_POINT('Origin',(-0.804195414779836,5.6,-9.14051516052749)) ;
#21848=CARTESIAN_POINT('Origin',(-2.6568964911086,5.6,-8.80800210238025)) ;
#21849=CARTESIAN_POINT('Origin',(0.172029571164298,5.6,-9.19839148039727)) ;
#21850=CARTESIAN_POINT('Origin',(-1.25767319645268,5.6,-9.11363034860009)) ;
#21851=CARTESIAN_POINT('',(-0.493406095500262,5.6,-8.32249458376462)) ;
#21852=CARTESIAN_POINT('Origin',(-0.54282181264419,5.6,-9.15601091449868)) ;
#21853=CARTESIAN_POINT('Origin',(0.172029571164298,5.6,-9.19839148039727)) ;
#21854=CARTESIAN_POINT('Origin',(1.59756323453576,5.6,-9.06023132771231)) ;
#21855=CARTESIAN_POINT('',(0.575602485190727,4.73397459621556,-8.65329616482006)) ;
#21856=CARTESIAN_POINT('',(0.672767480349251,4.73397459621556,-9.65584262129112)) ;
#21857=CARTESIAN_POINT('Origin',(0.624184982769988,5.6,-9.15456939305559)) ;
#21858=CARTESIAN_POINT('Origin',(1.59756323453576,4.73397459621556,-9.06023132771231)) ;
#21859=CARTESIAN_POINT('Origin',(1.59756323453576,4.7,-9.06023132771231)) ;
#21860=CARTESIAN_POINT('Ctrl Pts',(0.575602485190727,4.73397459621556,-8.65329616482006)) ;
#21861=CARTESIAN_POINT('Ctrl Pts',(0.553015540493783,4.68774565211319,-8.71002011751032)) ;
#21862=CARTESIAN_POINT('Ctrl Pts',(0.532688177667106,4.64764400859375,-8.77533191459035)) ;
#21863=CARTESIAN_POINT('Ctrl Pts',(0.498486784318542,4.57385160754098,-8.94720997429785)) ;
#21864=CARTESIAN_POINT('Ctrl Pts',(0.492356730589572,4.55136544237033,-9.05969114282006)) ;
#21865=CARTESIAN_POINT('Ctrl Pts',(0.513029963662795,4.55136544237033,-9.27299714389119)) ;
#21866=CARTESIAN_POINT('Ctrl Pts',(0.540645980075106,4.57385160754098,-9.38220770413312)) ;
#21867=CARTESIAN_POINT('Ctrl Pts',(0.607217027453607,4.64764400859375,-9.5443190805591)) ;
#21868=CARTESIAN_POINT('Ctrl Pts',(0.639708063086502,4.68774565211319,-9.60451181368207)) ;
#21869=CARTESIAN_POINT('Ctrl Pts',(0.672767480349251,4.73397459621556,-9.65584262129112)) ;
#21870=CARTESIAN_POINT('Origin',(0.172029571164298,5.6,-9.19839148039727)) ;
#21871=CARTESIAN_POINT('Origin',(1.59756323453576,5.6,-9.06023132771231)) ;
#21872=CARTESIAN_POINT('',(0.965343734874546,5.6,-9.96039714812994)) ;
#21873=CARTESIAN_POINT('Origin',(0.884796402850027,5.6,-9.12931140405479)) ;
#21874=CARTESIAN_POINT('Origin',(0.172029571164298,5.6,-9.19839148039727)) ;
#21875=CARTESIAN_POINT('Origin',(0.172029571164298,5.6,-9.19839148039727)) ;
#21876=CARTESIAN_POINT('',(1.24204919246076,5.6,-10.1011971128789)) ;
#21877=CARTESIAN_POINT('',(1.04876645339937,5.6,-8.10690971722908)) ;
#21878=CARTESIAN_POINT('Origin',(1.14540782293007,5.6,-9.10405341505399)) ;
#21879=CARTESIAN_POINT('Origin',(1.14540782293007,5.6,-9.10405341505399)) ;
#21880=CARTESIAN_POINT('Origin',(1.59756323453576,5.6,-9.06023132771231)) ;
#21881=CARTESIAN_POINT('',(1.59756323453576,5.6,-10.1602313277123)) ;
#21882=CARTESIAN_POINT('Origin',(1.59756323453576,5.6,-9.06023132771231)) ;
#21883=CARTESIAN_POINT('',(1.59756323453576,5.6,-7.96023132771231)) ;
#21884=CARTESIAN_POINT('Origin',(1.59756323453576,5.6,-9.06023132771231)) ;
#21885=CARTESIAN_POINT('Origin',(1.59756323453576,5.6,-9.06023132771231)) ;
#21886=CARTESIAN_POINT('',(0.720826352300685,5.6,-10.1517130908805)) ;
#21887=CARTESIAN_POINT('',(0.527543613239291,5.6,-8.15742569523067)) ;
#21888=CARTESIAN_POINT('Origin',(0.624184982769988,5.6,-9.15456939305559)) ;
#21889=CARTESIAN_POINT('Origin',(1.59756323453576,5.6,-9.06023132771231)) ;
#21890=CARTESIAN_POINT('Origin',(0.172029571164298,5.6,-9.19839148039727)) ;
#21891=CARTESIAN_POINT('',(-0.3407376054655,5.6,-10.1715666047049)) ;
#21892=CARTESIAN_POINT('',(-0.222158815551588,5.6,-8.17144673223487)) ;
#21893=CARTESIAN_POINT('Origin',(-0.281448210508544,5.6,-9.17150666846987)) ;
#21894=CARTESIAN_POINT('',(0.172029571164298,5.6,-10.2983914803973)) ;
#21895=CARTESIAN_POINT('Origin',(0.172029571164298,5.6,-9.19839148039727)) ;
#21896=CARTESIAN_POINT('Origin',(-0.281448210508544,5.6,-9.17150666846987)) ;
#21897=CARTESIAN_POINT('',(0.172029571164298,5.6,-8.09839148039727)) ;
#21898=CARTESIAN_POINT('Origin',(0.172029571164298,5.6,-9.19839148039727)) ;
#21899=CARTESIAN_POINT('Ctrl Pts',(0.720826352300685,5.6,-10.1517130908805)) ;
#21900=CARTESIAN_POINT('Ctrl Pts',(0.720826352300685,5.46171298397554,-10.1517130908805)) ;
#21901=CARTESIAN_POINT('Ctrl Pts',(0.696942796966399,5.31515492335585,-10.1336930651236)) ;
#21902=CARTESIAN_POINT('Ctrl Pts',(0.610345858722663,5.04666004644025,-10.0546352509191)) ;
#21903=CARTESIAN_POINT('Ctrl Pts',(0.548731949615678,4.9246088023834,-9.99278769580368)) ;
#21904=CARTESIAN_POINT('Ctrl Pts',(0.4274343396663,4.72890627139334,-9.8353688728735)) ;
#21905=CARTESIAN_POINT('Ctrl Pts',(0.359931166240814,4.64330837318027,-9.72855935219282)) ;
#21906=CARTESIAN_POINT('Ctrl Pts',(0.280974043242848,4.55782771698258,-9.54105603524641)) ;
#21907=CARTESIAN_POINT('Ctrl Pts',(0.258247910206437,4.53613333814489,-9.47410958337475)) ;
#21908=CARTESIAN_POINT('Ctrl Pts',(0.223193451378181,4.50745592650039,-9.33621765108249)) ;
#21909=CARTESIAN_POINT('Ctrl Pts',(0.210875366085843,4.50047177654324,-9.26526979989045)) ;
#21910=CARTESIAN_POINT('Ctrl Pts',(0.197309571397666,4.50047177654324,-9.12529820444441)) ;
#21911=CARTESIAN_POINT('Ctrl Pts',(0.195774098471602,4.50745592650039,-9.05330532190086)) ;
#21912=CARTESIAN_POINT('Ctrl Pts',(0.203696395774903,4.53613333814489,-8.91124815988333)) ;
#21913=CARTESIAN_POINT('Ctrl Pts',(0.213143660829931,4.55782771698258,-8.84118352027124)) ;
#21914=CARTESIAN_POINT('Ctrl Pts',(0.254624526417109,4.64330837318027,-8.64200757059819)) ;
#21915=CARTESIAN_POINT('Ctrl Pts',(0.300360457056649,4.72890627139334,-8.52422312010033)) ;
#21916=CARTESIAN_POINT('Ctrl Pts',(0.389170995352308,4.9246088023834,-8.3464409942277)) ;
#21917=CARTESIAN_POINT('Ctrl Pts',(0.437761432854958,5.04666004644025,-8.27391263251655)) ;
#21918=CARTESIAN_POINT('Ctrl Pts',(0.507564998098324,5.31515492335585,-8.17969676347481)) ;
#21919=CARTESIAN_POINT('Ctrl Pts',(0.527543613239291,5.46171298397554,-8.15742569523067)) ;
#21920=CARTESIAN_POINT('Ctrl Pts',(0.527543613239291,5.6,-8.15742569523067)) ;
#21921=CARTESIAN_POINT('Origin',(1.59756323453576,4.7,-9.06023132771231)) ;
#21922=CARTESIAN_POINT('Origin',(-1.25767319645268,5.6,-9.11363034860009)) ;
#21923=CARTESIAN_POINT('Origin',(-1.25767319645268,5.6,-9.11363034860009)) ;
#21924=CARTESIAN_POINT('',(-1.25767319645267,7.,-9.11363034860001)) ;
#21925=CARTESIAN_POINT('',(-1.34052789309705,5.6,-10.5111764477481)) ;
#21926=CARTESIAN_POINT('Origin',(-1.25767319645268,5.6,-9.11363034860008)) ;
#21927=CARTESIAN_POINT('',(-1.25767319645267,4.2,-9.11363034860001)) ;
#21928=CARTESIAN_POINT('Origin',(-1.25767319645268,5.6,-9.11363034860008)) ;
#21929=CARTESIAN_POINT('',(-1.55642729623381,5.6,-10.4813825146974)) ;
#21930=CARTESIAN_POINT('Origin',(-1.25767319645268,5.6,-9.11363034860009)) ;
#21931=CARTESIAN_POINT('Origin',(-1.25767319645268,5.6,-9.11363034860009)) ;
#21932=CARTESIAN_POINT('Origin',(-2.6568964911086,5.6,-8.80800210238025)) ;
#21933=CARTESIAN_POINT('',(-2.6568964911086,7.,-8.80800210238028)) ;
#21934=CARTESIAN_POINT('',(-2.95565059088973,5.6,-10.1757542684776)) ;
#21935=CARTESIAN_POINT('Origin',(-2.6568964911086,5.6,-8.80800210238025)) ;
#21936=CARTESIAN_POINT('',(-2.6568964911086,4.2,-8.80800210238028)) ;
#21937=CARTESIAN_POINT('Origin',(-2.6568964911086,5.6,-8.80800210238025)) ;
#21938=CARTESIAN_POINT('',(-3.16430974470577,5.6,-10.1128131193762)) ;
#21939=CARTESIAN_POINT('Origin',(-2.6568964911086,5.6,-8.80800210238025)) ;
#21940=CARTESIAN_POINT('Origin',(-2.6568964911086,5.6,-8.80800210238025)) ;
#21941=CARTESIAN_POINT('Origin',(-6.34117671405231,5.6,-6.66554407990531)) ;
#21942=CARTESIAN_POINT('',(-6.34117671405228,7.,-6.66554407990528)) ;
#21943=CARTESIAN_POINT('',(-7.22425828324403,5.6,-7.75189896766248)) ;
#21944=CARTESIAN_POINT('Origin',(-6.34117671405231,5.6,-6.66554407990531)) ;
#21945=CARTESIAN_POINT('',(-6.34117671405228,4.2,-6.66554407990528)) ;
#21946=CARTESIAN_POINT('Origin',(-6.34117671405231,5.6,-6.66554407990531)) ;
#21947=CARTESIAN_POINT('',(-7.38216319417279,5.6,-7.60167823065849)) ;
#21948=CARTESIAN_POINT('Origin',(-6.34117671405231,5.6,-6.66554407990531)) ;
#21949=CARTESIAN_POINT('Origin',(-6.34117671405231,5.6,-6.66554407990531)) ;
#21950=CARTESIAN_POINT('Origin',(-7.29885073067936,5.6,-5.60060514688023)) ;
#21951=CARTESIAN_POINT('',(-7.29885073067936,7.,-5.60060514688023)) ;
#21952=CARTESIAN_POINT('',(-8.33983721079984,5.6,-6.53673929763341)) ;
#21953=CARTESIAN_POINT('Origin',(-7.29885073067936,5.6,-5.60060514688023)) ;
#21954=CARTESIAN_POINT('',(-7.29885073067936,4.2,-5.60060514688023)) ;
#21955=CARTESIAN_POINT('Origin',(-7.29885073067936,5.6,-5.60060514688023)) ;
#21956=CARTESIAN_POINT('',(-8.47251401051246,5.6,-6.36383152586056)) ;
#21957=CARTESIAN_POINT('Origin',(-7.29885073067936,5.6,-5.60060514688023)) ;
#21958=CARTESIAN_POINT('Origin',(-7.29885073067936,5.6,-5.60060514688023)) ;
#21959=CARTESIAN_POINT('Origin',(-9.03961155374625,5.6,-1.71038678589882)) ;
#21960=CARTESIAN_POINT('',(-9.03961155374629,7.,-1.71038678589883)) ;
#21961=CARTESIAN_POINT('',(-10.3907718334498,5.6,-2.0769463288812)) ;
#21962=CARTESIAN_POINT('Origin',(-9.03961155374625,5.6,-1.71038678589882)) ;
#21963=CARTESIAN_POINT('',(-9.03961155374629,4.2,-1.71038678589883)) ;
#21964=CARTESIAN_POINT('Origin',(-9.03961155374625,5.6,-1.71038678589882)) ;
#21965=CARTESIAN_POINT('',(-10.4312904272575,5.6,-1.86280041069157)) ;
#21966=CARTESIAN_POINT('Origin',(-9.03961155374625,5.6,-1.71038678589882)) ;
#21967=CARTESIAN_POINT('Origin',(-9.03961155374625,5.6,-1.71038678589882)) ;
#21968=CARTESIAN_POINT('Origin',(-9.19553212146245,5.6,-0.286686245139542)) ;
#21969=CARTESIAN_POINT('',(-9.19553212146238,7.,-0.286686245139535)) ;
#21970=CARTESIAN_POINT('',(-10.5872109949737,5.6,-0.439099869932289)) ;
#21971=CARTESIAN_POINT('Origin',(-9.19553212146245,5.6,-0.286686245139542)) ;
#21972=CARTESIAN_POINT('',(-9.19553212146238,4.2,-0.286686245139535)) ;
#21973=CARTESIAN_POINT('Origin',(-9.19553212146245,5.6,-0.286686245139542)) ;
#21974=CARTESIAN_POINT('',(-10.5940025134845,5.6,-0.221260236261659)) ;
#21975=CARTESIAN_POINT('Origin',(-9.19553212146245,5.6,-0.286686245139543)) ;
#21976=CARTESIAN_POINT('Origin',(-9.19553212146245,5.6,-0.286686245139543)) ;
#21977=CARTESIAN_POINT('Origin',(-8.33803164073718,5.6,3.88808800801444)) ;
#21978=CARTESIAN_POINT('',(-9.36813072379435,4.73397459621556,4.27395829591541)) ;
#21979=CARTESIAN_POINT('',(-7.30793255768001,4.73397459621556,3.50221772011346)) ;
#21980=CARTESIAN_POINT('Origin',(-8.33803164073718,5.6,3.88808800801444)) ;
#21981=CARTESIAN_POINT('Origin',(-8.33803164073718,4.73397459621556,3.88808800801444)) ;
#21982=CARTESIAN_POINT('Origin',(-8.33803164073718,5.6,3.88808800801444)) ;
#21983=CARTESIAN_POINT('',(-7.02699644411896,5.6,3.39698036886774)) ;
#21984=CARTESIAN_POINT('',(-7.07983245007737,5.9934418358376,3.41677248902982)) ;
#21985=CARTESIAN_POINT('Origin',(-8.33803164073718,5.6,3.88808800801444)) ;
#21986=CARTESIAN_POINT('',(-7.5297412638717,6.40829037686548,4.69637838487991)) ;
#21987=CARTESIAN_POINT('Origin',(-8.33803164073718,5.6,3.88808800801444)) ;
#21988=CARTESIAN_POINT('',(-9.64906683735539,5.6,4.37919564716113)) ;
#21989=CARTESIAN_POINT('Origin',(-8.33803164073718,5.6,3.88808800801444)) ;
#21990=CARTESIAN_POINT('Origin',(-8.33803164073718,5.6,3.88808800801444)) ;
#21991=CARTESIAN_POINT('Origin',(-8.33803164073718,4.7,3.88808800801444)) ;
#21992=CARTESIAN_POINT('',(-9.43803164073718,3.8,3.88808800801444)) ;
#21993=CARTESIAN_POINT('Origin',(-8.33803164073718,3.8,3.88808800801444)) ;
#21994=CARTESIAN_POINT('',(-9.43803164073718,4.65189880335233,3.88808800801446)) ;
#21995=CARTESIAN_POINT('',(-9.43803164073718,4.7,3.88808800801444)) ;
#21996=CARTESIAN_POINT('Ctrl Pts',(-9.43803164073718,4.65189880335233,3.88808800801448)) ;
#21997=CARTESIAN_POINT('Ctrl Pts',(-9.43803164073718,4.67348663571234,3.94472968162414)) ;
#21998=CARTESIAN_POINT('Ctrl Pts',(-9.43364416512203,4.6921524379,4.00185692423036)) ;
#21999=CARTESIAN_POINT('Ctrl Pts',(-9.41328552009356,4.72400374275534,4.13153241586434)) ;
#22000=CARTESIAN_POINT('Ctrl Pts',(-9.39435951087235,4.73397459621556,4.20393930153851)) ;
#22001=CARTESIAN_POINT('Ctrl Pts',(-9.36813072379435,4.73397459621556,4.27395829591541)) ;
#22002=CARTESIAN_POINT('Ctrl Pts',(-7.30793255768001,4.73397459621556,3.50221772011346)) ;
#22003=CARTESIAN_POINT('Ctrl Pts',(-7.33416134475801,4.73397459621556,3.43219872573657)) ;
#22004=CARTESIAN_POINT('Ctrl Pts',(-7.36746447425383,4.72400374275534,3.3651774419242)) ;
#22005=CARTESIAN_POINT('Ctrl Pts',(-7.4459311319277,4.68822251881602,3.24032819717562)) ;
#22006=CARTESIAN_POINT('Ctrl Pts',(-7.49109925396746,4.66259261868094,3.1824514714858)) ;
#22007=CARTESIAN_POINT('Ctrl Pts',(-7.64041858377118,4.57386929426243,3.02541433890689)) ;
#22008=CARTESIAN_POINT('Ctrl Pts',(-7.7594241100859,4.49983982293173,2.94283961099156)) ;
#22009=CARTESIAN_POINT('Ctrl Pts',(-8.00214210356859,4.37384612030215,2.83240931234868)) ;
#22010=CARTESIAN_POINT('Ctrl Pts',(-8.14325908220336,4.31153832429548,2.79560182561931)) ;
#22011=CARTESIAN_POINT('Ctrl Pts',(-8.36279722995668,4.24614166874784,2.78592998438068)) ;
#22012=CARTESIAN_POINT('Ctrl Pts',(-8.43733422265602,4.22885243350374,2.79007110227452)) ;
#22013=CARTESIAN_POINT('Ctrl Pts',(-8.58385009380069,4.20577546283643,2.81334365875814)) ;
#22014=CARTESIAN_POINT('Ctrl Pts',(-8.65582869467146,4.2,2.83248901060814)) ;
#22015=CARTESIAN_POINT('Ctrl Pts',(-8.79197516260484,4.2,2.88348883930639)) ;
#22016=CARTESIAN_POINT('Ctrl Pts',(-8.8588176742847,4.20577546283643,2.91634522549083)) ;
#22017=CARTESIAN_POINT('Ctrl Pts',(-8.984564742228,4.22885243350374,2.99506108975102)) ;
#22018=CARTESIAN_POINT('Ctrl Pts',(-9.04347823023389,4.24614166874784,3.04090989637728)) ;
#22019=CARTESIAN_POINT('Ctrl Pts',(-9.20263169412595,4.31153832429548,3.19243784021295)) ;
#22020=CARTESIAN_POINT('Ctrl Pts',(-9.28483603338533,4.37384612030215,3.31290044580185)) ;
#22021=CARTESIAN_POINT('Ctrl Pts',(-9.39526633202821,4.49983982293173,3.55561843928454)) ;
#22022=CARTESIAN_POINT('Ctrl Pts',(-9.43073199452746,4.57386929426243,3.69605735044247)) ;
#22023=CARTESIAN_POINT('Ctrl Pts',(-9.43768488048529,4.63951461020542,3.85623687470378)) ;
#22024=CARTESIAN_POINT('Ctrl Pts',(-9.43803164073718,4.64582185322758,3.87214344166024)) ;
#22025=CARTESIAN_POINT('Ctrl Pts',(-9.43803164073718,4.65189880335233,3.88808800801448)) ;
#22026=CARTESIAN_POINT('Origin',(1.59756323453576,4.7,-9.06023132771231)) ;
#22027=CARTESIAN_POINT('',(0.197563234535756,3.8,-9.06023132771231)) ;
#22028=CARTESIAN_POINT('Origin',(1.59756323453576,3.8,-9.06023132771231)) ;
#22029=CARTESIAN_POINT('',(0.197563234535756,4.206529234206,-9.06023132771231)) ;
#22030=CARTESIAN_POINT('',(0.197563234535756,4.7,-9.06023132771231)) ;
#22031=CARTESIAN_POINT('',(1.73261590899087,5.6,-10.4537020935063)) ;
#22032=CARTESIAN_POINT('Origin',(1.59756323453576,5.6,-9.06023132771231)) ;
#22033=CARTESIAN_POINT('',(2.58751272819692,5.6,-10.0501808213735)) ;
#22034=CARTESIAN_POINT('Origin',(1.59756323453576,5.6,-9.06023132771231)) ;
#22035=CARTESIAN_POINT('',(1.46251056008064,5.6,-7.66676056191831)) ;
#22036=CARTESIAN_POINT('Origin',(1.59756323453576,5.6,-9.06023132771231)) ;
#22037=CARTESIAN_POINT('Origin',(1.59756323453576,5.6,-9.06023132771231)) ;
#22038=CARTESIAN_POINT('Origin',(1.59756323453576,3.8,-9.06023132771231)) ;
#22039=CARTESIAN_POINT('',(0.497563234535756,3.8,-9.06023132771231)) ;
#22040=CARTESIAN_POINT('Origin',(1.59756323453576,3.8,-9.06023132771231)) ;
#22041=CARTESIAN_POINT('Origin',(0.884796402850027,5.6,-9.12931140405479)) ;
#22042=CARTESIAN_POINT('',(0.145771492360773,5.6,-7.7943765385289)) ;
#22043=CARTESIAN_POINT('',(0.749743728394908,5.6,-7.73584063826079)) ;
#22044=CARTESIAN_POINT('',(0.172029571164301,4.2,-9.1983914803973)) ;
#22045=CARTESIAN_POINT('Origin',(0.172029571164302,5.6,-9.19839148039727)) ;
#22046=CARTESIAN_POINT('',(0.172029571164301,7.,-9.1983914803973)) ;
#22047=CARTESIAN_POINT('Origin',(0.172029571164298,5.6,-9.19839148039727)) ;
#22048=CARTESIAN_POINT('Origin',(0.172029571164302,5.6,-9.19839148039727)) ;
#22049=CARTESIAN_POINT('Origin',(1.59756323453576,5.6,-9.06023132771231)) ;
#22050=CARTESIAN_POINT('Origin',(0.884796402850027,5.6,-9.12931140405479)) ;
#22051=CARTESIAN_POINT('',(1.49145041889245,4.73397459621556,-7.96536144030274)) ;
#22052=CARTESIAN_POINT('',(0.497563234535756,4.20402719569605,-9.06023132771226)) ;
#22053=CARTESIAN_POINT('Ctrl Pts',(1.49145041889245,4.73397459621556,-7.96536144030274)) ;
#22054=CARTESIAN_POINT('Ctrl Pts',(1.41702875426729,4.73397459621556,-7.97257425386995)) ;
#22055=CARTESIAN_POINT('Ctrl Pts',(1.34367168114684,4.72400374275534,-7.98739622206835)) ;
#22056=CARTESIAN_POINT('Ctrl Pts',(1.20276790583996,4.68822251881602,-8.03087583091053)) ;
#22057=CARTESIAN_POINT('Ctrl Pts',(1.13517291153972,4.66259261868094,-8.05952528763701)) ;
#22058=CARTESIAN_POINT('Ctrl Pts',(0.944840003140219,4.57386929426243,-8.16311248395889)) ;
#22059=CARTESIAN_POINT('Ctrl Pts',(0.834278044165309,4.49983982293173,-8.25669108306875)) ;
#22060=CARTESIAN_POINT('Ctrl Pts',(0.664790527398948,4.37384612030215,-8.4625571970336)) ;
#22061=CARTESIAN_POINT('Ctrl Pts',(0.592713463708253,4.31153832429548,-8.58933925265689)) ;
#22062=CARTESIAN_POINT('Ctrl Pts',(0.526550528703005,4.24614166874784,-8.79889356271373)) ;
#22063=CARTESIAN_POINT('Ctrl Pts',(0.511258948151115,4.22885243350373,-8.87196256915488)) ;
#22064=CARTESIAN_POINT('Ctrl Pts',(0.499550081017094,4.21135383689655,-8.98384305616054)) ;
#22065=CARTESIAN_POINT('Ctrl Pts',(0.497563234535756,4.20690935315874,-9.02213729089606)) ;
#22066=CARTESIAN_POINT('Ctrl Pts',(0.497563234535756,4.20402719569605,-9.0602313277122)) ;
#22067=CARTESIAN_POINT('',(1.70367605017906,4.73397459621556,-10.1551012151219)) ;
#22068=CARTESIAN_POINT('Ctrl Pts',(0.497563234535756,4.20402719569605,-9.0602313277122)) ;
#22069=CARTESIAN_POINT('Ctrl Pts',(0.497563234535756,4.201329636592,-9.09588549205045)) ;
#22070=CARTESIAN_POINT('Ctrl Pts',(0.499303157025686,4.2,-9.1313642304099)) ;
#22071=CARTESIAN_POINT('Ctrl Pts',(0.509705723551869,4.2,-9.2386977016051)) ;
#22072=CARTESIAN_POINT('Ctrl Pts',(0.524142440480705,4.20577546283643,-9.31176646842849)) ;
#22073=CARTESIAN_POINT('Ctrl Pts',(0.567630390658757,4.22885243350374,-9.45360197375729)) ;
#22074=CARTESIAN_POINT('Ctrl Pts',(0.596669004374252,4.24614166874784,-9.52237457768905)) ;
#22075=CARTESIAN_POINT('Ctrl Pts',(0.701841811180312,4.31153832429548,-9.71532333653564)) ;
#22076=CARTESIAN_POINT('Ctrl Pts',(0.796923704430307,4.37384612030215,-9.82590464740839)) ;
#22077=CARTESIAN_POINT('Ctrl Pts',(1.00278981839516,4.49983982293173,-9.99539216417475)) ;
#22078=CARTESIAN_POINT('Ctrl Pts',(1.12926420079653,4.57386929426243,-10.0659976284104)) ;
#22079=CARTESIAN_POINT('Ctrl Pts',(1.33594685627334,4.66259261868093,-10.1311067920257)) ;
#22080=CARTESIAN_POINT('Ctrl Pts',(1.40778543927975,4.68822251881602,-10.1462425978121)) ;
#22081=CARTESIAN_POINT('Ctrl Pts',(1.55441629304583,4.72400374275534,-10.1618548687754)) ;
#22082=CARTESIAN_POINT('Ctrl Pts',(1.62925438555391,4.73397459621556,-10.1623140286891)) ;
#22083=CARTESIAN_POINT('Ctrl Pts',(1.70367605017906,4.73397459621556,-10.1551012151219)) ;
#22084=CARTESIAN_POINT('Origin',(1.59756323453576,5.6,-9.06023132771231)) ;
#22085=CARTESIAN_POINT('Origin',(-0.54282181264419,5.6,-9.15601091449868)) ;
#22086=CARTESIAN_POINT('',(0.0891748745199313,5.6,-10.5959375795453)) ;
#22087=CARTESIAN_POINT('Origin',(0.172029571164298,5.6,-9.19839148039727)) ;
#22088=CARTESIAN_POINT('',(-0.625676509288564,5.6,-10.5535570136467)) ;
#22089=CARTESIAN_POINT('Origin',(-1.25767319645268,5.6,-9.11363034860008)) ;
#22090=CARTESIAN_POINT('Origin',(0.172029571164298,5.6,-9.19839148039727)) ;
#22091=CARTESIAN_POINT('Origin',(-1.95728484378064,5.6,-8.96081622549017)) ;
#22092=CARTESIAN_POINT('',(-2.25603894356177,5.6,-10.3285683915875)) ;
#22093=CARTESIAN_POINT('Origin',(-2.65689649110859,5.6,-8.80800210238025)) ;
#22094=CARTESIAN_POINT('Origin',(-3.32431344549507,5.6,-8.54845784354125)) ;
#22095=CARTESIAN_POINT('',(-4.49914365347872,5.6,-9.59372460169817)) ;
#22096=CARTESIAN_POINT('',(-3.83172669909225,5.6,-9.85326886053717)) ;
#22097=CARTESIAN_POINT('',(-3.99173039988151,7.,-8.2889135847022)) ;
#22098=CARTESIAN_POINT('Origin',(-3.99173039988154,5.6,-8.28891358470225)) ;
#22099=CARTESIAN_POINT('',(-3.99173039988151,4.2,-8.2889135847022)) ;
#22100=CARTESIAN_POINT('Origin',(-3.99173039988154,5.6,-8.28891358470225)) ;
#22101=CARTESIAN_POINT('Origin',(-3.99173039988154,5.6,-8.28891358470225)) ;
#22102=CARTESIAN_POINT('Origin',(-4.61077793718327,5.6,-7.92892919634708)) ;
#22103=CARTESIAN_POINT('',(-4.69550574269427,5.6,-9.49916160343595)) ;
#22104=CARTESIAN_POINT('Origin',(-3.99173039988154,5.6,-8.28891358470226)) ;
#22105=CARTESIAN_POINT('',(-5.93360081729775,5.6,-8.7791928267256)) ;
#22106=CARTESIAN_POINT('',(-5.31455327999601,5.6,-9.13917721508077)) ;
#22107=CARTESIAN_POINT('',(-5.22982547448502,7.,-7.56894480799192)) ;
#22108=CARTESIAN_POINT('Origin',(-5.22982547448501,5.6,-7.56894480799191)) ;
#22109=CARTESIAN_POINT('',(-5.22982547448502,4.2,-7.56894480799192)) ;
#22110=CARTESIAN_POINT('Origin',(-5.22982547448501,5.6,-7.56894480799191)) ;
#22111=CARTESIAN_POINT('Origin',(-5.22982547448501,5.6,-7.56894480799191)) ;
#22112=CARTESIAN_POINT('Origin',(-3.99173039988154,5.6,-8.28891358470226)) ;
#22113=CARTESIAN_POINT('Origin',(-5.78550109426866,5.6,-7.11724444394861)) ;
#22114=CARTESIAN_POINT('',(-6.11290704367673,5.6,-8.65529969574907)) ;
#22115=CARTESIAN_POINT('Origin',(-5.22982547448501,5.6,-7.56894480799191)) ;
#22116=CARTESIAN_POINT('',(-6.66858266346038,5.6,-8.20359933170578)) ;
#22117=CARTESIAN_POINT('Origin',(-6.34117671405231,5.6,-6.66554407990531)) ;
#22118=CARTESIAN_POINT('Origin',(-5.22982547448501,5.6,-7.56894480799191)) ;
#22119=CARTESIAN_POINT('Origin',(-6.82001372236584,5.6,-6.13307461339277)) ;
#22120=CARTESIAN_POINT('',(-7.86100020248631,5.6,-7.06920876414595)) ;
#22121=CARTESIAN_POINT('Origin',(-7.29885073067936,5.6,-5.60060514688023)) ;
#22122=CARTESIAN_POINT('Origin',(-7.68924460284273,5.6,-5.00027087509818)) ;
#22123=CARTESIAN_POINT('',(-9.2533017548392,5.6,-5.16316298229645)) ;
#22124=CARTESIAN_POINT('',(-8.86290788267583,5.6,-5.7634972540785)) ;
#22125=CARTESIAN_POINT('',(-8.0796384750061,7.,-4.39993660331612)) ;
#22126=CARTESIAN_POINT('Origin',(-8.0796384750061,5.6,-4.39993660331612)) ;
#22127=CARTESIAN_POINT('',(-8.0796384750061,4.2,-4.39993660331612)) ;
#22128=CARTESIAN_POINT('Origin',(-8.0796384750061,5.6,-4.39993660331613)) ;
#22129=CARTESIAN_POINT('Origin',(-8.0796384750061,5.6,-4.39993660331612)) ;
#22130=CARTESIAN_POINT('Origin',(-8.37212808908055,5.6,-3.74628651423376)) ;
#22131=CARTESIAN_POINT('',(-9.35753504609195,5.6,-4.97175856302653)) ;
#22132=CARTESIAN_POINT('Origin',(-8.0796384750061,5.6,-4.39993660331612)) ;
#22133=CARTESIAN_POINT('',(-9.94251427424083,5.6,-3.6644583848618)) ;
#22134=CARTESIAN_POINT('',(-9.65002466016639,5.6,-4.31810847394416)) ;
#22135=CARTESIAN_POINT('',(-8.66461770315502,7.,-3.09263642515142)) ;
#22136=CARTESIAN_POINT('Origin',(-8.66461770315499,5.6,-3.0926364251514)) ;
#22137=CARTESIAN_POINT('',(-8.66461770315502,4.2,-3.09263642515142)) ;
#22138=CARTESIAN_POINT('Origin',(-8.66461770315498,5.6,-3.09263642515141)) ;
#22139=CARTESIAN_POINT('Origin',(-8.66461770315499,5.6,-3.0926364251514)) ;
#22140=CARTESIAN_POINT('Origin',(-8.0796384750061,5.6,-4.39993660331612)) ;
#22141=CARTESIAN_POINT('Origin',(-8.85211462845062,5.6,-2.40151160552511)) ;
#22142=CARTESIAN_POINT('',(-10.0157779828585,5.6,-3.45919596813381)) ;
#22143=CARTESIAN_POINT('Origin',(-8.66461770315498,5.6,-3.0926364251514)) ;
#22144=CARTESIAN_POINT('',(-10.2032749081542,5.6,-2.7680711485075)) ;
#22145=CARTESIAN_POINT('Origin',(-9.03961155374625,5.6,-1.71038678589882)) ;
#22146=CARTESIAN_POINT('Origin',(-8.66461770315498,5.6,-3.0926364251514)) ;
#22147=CARTESIAN_POINT('Origin',(-9.11757183760435,5.6,-0.998536515519179)) ;
#22148=CARTESIAN_POINT('',(-10.5092507111156,5.6,-1.15095014031193)) ;
#22149=CARTESIAN_POINT('Origin',(-9.19553212146245,5.6,-0.286686245139533)) ;
#22150=CARTESIAN_POINT('Origin',(-9.16206641109202,5.6,0.428637918808661)) ;
#22151=CARTESIAN_POINT('',(-10.5270710927436,5.6,1.20938809163475)) ;
#22152=CARTESIAN_POINT('',(-10.5605368031141,5.6,0.494063927686545)) ;
#22153=CARTESIAN_POINT('',(-9.12860070072155,7.,1.14396208275686)) ;
#22154=CARTESIAN_POINT('Origin',(-9.12860070072158,5.6,1.14396208275687)) ;
#22155=CARTESIAN_POINT('',(-9.12860070072155,4.2,1.14396208275686)) ;
#22156=CARTESIAN_POINT('Origin',(-9.12860070072158,5.6,1.14396208275685)) ;
#22157=CARTESIAN_POINT('Origin',(-9.12860070072158,5.6,1.14396208275687)) ;
#22158=CARTESIAN_POINT('Origin',(-8.98452003130825,5.6,1.84542439393274)) ;
#22159=CARTESIAN_POINT('',(-10.499970944786,5.6,1.42564213830696)) ;
#22160=CARTESIAN_POINT('Origin',(-9.12860070072158,5.6,1.14396208275687)) ;
#22161=CARTESIAN_POINT('',(-10.2118096059593,5.6,2.82856676065872)) ;
#22162=CARTESIAN_POINT('',(-10.3558902753727,5.6,2.12710444948285)) ;
#22163=CARTESIAN_POINT('',(-8.84043936189494,7.,2.54688670510862)) ;
#22164=CARTESIAN_POINT('Origin',(-8.84043936189492,5.6,2.54688670510862)) ;
#22165=CARTESIAN_POINT('',(-8.84043936189494,4.2,2.54688670510862)) ;
#22166=CARTESIAN_POINT('Origin',(-8.84043936189492,5.6,2.54688670510861)) ;
#22167=CARTESIAN_POINT('Origin',(-8.84043936189492,5.6,2.54688670510862)) ;
#22168=CARTESIAN_POINT('Origin',(-9.12860070072158,5.6,1.14396208275687)) ;
#22169=CARTESIAN_POINT('Origin',(-8.58923550131605,5.6,3.21748735656153)) ;
#22170=CARTESIAN_POINT('',(-10.1514745585131,5.6,3.0379943442553)) ;
#22171=CARTESIAN_POINT('Origin',(-8.84043936189492,5.6,2.54688670510862)) ;
#22172=CARTESIAN_POINT('',(-9.90027069793426,5.6,3.70859499570822)) ;
#22173=CARTESIAN_POINT('',(-9.73803164073718,5.10889236085331,3.88808800801444)) ;
#22174=CARTESIAN_POINT('Origin',(-8.33803164073718,5.6,3.88808800801444)) ;
#22175=CARTESIAN_POINT('Origin',(-8.33803164073718,5.6,3.88808800801444)) ;
#22176=CARTESIAN_POINT('Origin',(-8.84043936189492,5.6,2.54688670510862)) ;
#22177=CARTESIAN_POINT('Origin',(-8.58923550131605,5.6,3.21748735656153)) ;
#22178=CARTESIAN_POINT('Origin',(-8.33803164073718,4.7,3.88808800801444)) ;
#22179=CARTESIAN_POINT('',(-9.73803164073718,3.8,3.88808800801444)) ;
#22180=CARTESIAN_POINT('',(-9.73803164073718,4.7,3.88808800801444)) ;
#22181=CARTESIAN_POINT('Origin',(-8.33803164073718,3.8,3.88808800801444)) ;
#22182=CARTESIAN_POINT('Origin',(-8.33803164073718,3.8,3.88808800801444)) ;
#22183=CARTESIAN_POINT('Origin',(-8.84043936189492,5.6,2.54688670510862)) ;
#22184=CARTESIAN_POINT('Origin',(-9.12860070072158,5.6,1.14396208275687)) ;
#22185=CARTESIAN_POINT('Origin',(-8.66461770315499,5.6,-3.0926364251514)) ;
#22186=CARTESIAN_POINT('Origin',(-8.0796384750061,5.6,-4.39993660331612)) ;
#22187=CARTESIAN_POINT('Origin',(-5.22982547448501,5.6,-7.56894480799191)) ;
#22188=CARTESIAN_POINT('Origin',(-3.99173039988154,5.6,-8.28891358470226)) ;
#22189=CARTESIAN_POINT('Origin',(0.172029571164298,5.6,-9.19839148039727)) ;
#22190=CARTESIAN_POINT('',(0.172029571164298,5.6,-10.5983914803973)) ;
#22191=CARTESIAN_POINT('Origin',(0.172029571164298,5.6,-9.19839148039727)) ;
#22192=CARTESIAN_POINT('Origin',(1.59756323453576,4.7,-9.06023132771231)) ;
#22193=CARTESIAN_POINT('Origin',(1.59756323453576,4.73397459621556,-9.06023132771231)) ;
#22194=CARTESIAN_POINT('',(0.497563234535756,4.7,-9.06023132771231)) ;
#22195=CARTESIAN_POINT('Origin',(1.59756323453576,5.6,-9.06023132771231)) ;
#22196=CARTESIAN_POINT('',(2.40585361140123,6.40829037686548,-8.25194095084684)) ;
#22197=CARTESIAN_POINT('Origin',(1.59756323453576,5.6,-9.06023132771231)) ;
#22198=CARTESIAN_POINT('Origin',(1.59756323453576,5.6,-9.06023132771231)) ;
#22199=CARTESIAN_POINT('Origin',(-1.25767319645268,5.6,-9.11363034860009)) ;
#22200=CARTESIAN_POINT('',(-1.77910365806296,5.6,-8.14506941933188)) ;
#22201=CARTESIAN_POINT('Origin',(-1.95728484378064,5.6,-8.96081622549017)) ;
#22202=CARTESIAN_POINT('Origin',(-2.6568964911086,5.6,-8.80800210238025)) ;
#22203=CARTESIAN_POINT('Origin',(-3.99173039988154,5.6,-8.28891358470226)) ;
#22204=CARTESIAN_POINT('',(-4.61077793718327,4.76502012796642,-7.92892919634708)) ;
#22205=CARTESIAN_POINT('Origin',(-4.61077793718327,5.6,-7.92892919634708)) ;
#22206=CARTESIAN_POINT('Origin',(-5.22982547448501,5.6,-7.56894480799191)) ;
#22207=CARTESIAN_POINT('Origin',(-6.34117671405231,5.6,-6.66554407990531)) ;
#22208=CARTESIAN_POINT('',(-7.44087283519418,5.6,-6.69139830868002)) ;
#22209=CARTESIAN_POINT('Origin',(-6.82001372236584,5.6,-6.13307461339277)) ;
#22210=CARTESIAN_POINT('',(-6.34117671405231,5.6,-5.56554407990531)) ;
#22211=CARTESIAN_POINT('Origin',(-6.34117671405231,5.6,-6.66554407990531)) ;
#22212=CARTESIAN_POINT('Origin',(-7.29885073067936,5.6,-5.60060514688023)) ;
#22213=CARTESIAN_POINT('',(-7.29885073067936,5.6,-6.70060514688023)) ;
#22214=CARTESIAN_POINT('Origin',(-7.29885073067936,5.6,-5.60060514688023)) ;
#22215=CARTESIAN_POINT('Origin',(-8.0796384750061,5.6,-4.39993660331612)) ;
#22216=CARTESIAN_POINT('',(-9.13428374293583,5.6,-4.08732924762303)) ;
#22217=CARTESIAN_POINT('Origin',(-8.37212808908055,5.6,-3.74628651423376)) ;
#22218=CARTESIAN_POINT('',(-8.0796384750061,5.6,-3.29993660331612)) ;
#22219=CARTESIAN_POINT('Origin',(-8.0796384750061,5.6,-4.39993660331612)) ;
#22220=CARTESIAN_POINT('Origin',(-8.66461770315499,5.6,-3.0926364251514)) ;
#22221=CARTESIAN_POINT('',(-8.66461770315499,5.6,-4.1926364251514)) ;
#22222=CARTESIAN_POINT('Origin',(-8.66461770315499,5.6,-3.0926364251514)) ;
#22223=CARTESIAN_POINT('Origin',(-9.03961155374625,5.6,-1.71038678589882)) ;
#22224=CARTESIAN_POINT('',(-9.94758887168739,5.6,-1.08943816475177)) ;
#22225=CARTESIAN_POINT('Origin',(-9.11757183760435,5.6,-0.998536515519179)) ;
#22226=CARTESIAN_POINT('',(-9.03961155374625,5.6,-0.610386785898816)) ;
#22227=CARTESIAN_POINT('Origin',(-9.03961155374625,5.6,-1.71038678589882)) ;
#22228=CARTESIAN_POINT('Origin',(-9.19553212146245,5.6,-0.286686245139542)) ;
#22229=CARTESIAN_POINT('',(-9.19553212146245,5.6,-1.38668624513954)) ;
#22230=CARTESIAN_POINT('Origin',(-9.19553212146245,5.6,-0.286686245139542)) ;
#22231=CARTESIAN_POINT('Origin',(-9.12860070072158,5.6,1.14396208275687)) ;
#22232=CARTESIAN_POINT('',(-9.80242471052222,5.6,2.01342237731677)) ;
#22233=CARTESIAN_POINT('Origin',(-8.98452003130825,5.6,1.84542439393274)) ;
#22234=CARTESIAN_POINT('',(-9.12860070072158,5.6,2.24396208275687)) ;
#22235=CARTESIAN_POINT('Origin',(-9.12860070072158,5.6,1.14396208275687)) ;
#22236=CARTESIAN_POINT('Origin',(-8.84043936189492,5.6,2.54688670510862)) ;
#22237=CARTESIAN_POINT('',(-8.84043936189492,5.6,1.44688670510862)) ;
#22238=CARTESIAN_POINT('Origin',(-8.84043936189492,5.6,2.54688670510862)) ;
#24552=UNCERTAINTY_MEASURE_WITH_UNIT(LENGTH_MEASURE(0.001),#24629,
'DISTANCE_ACCURACY_VALUE',
'Maximum model space distance between geometric entities at asserted c
onnectivities') ;
#24580=UNCERTAINTY_MEASURE_WITH_UNIT(LENGTH_MEASURE(0.001),#24629,
'DISTANCE_ACCURACY_VALUE',
'Maximum model space distance between geometric entities at asserted c
onnectivities') ;
#24600=(
GEOMETRIC_REPRESENTATION_CONTEXT(3)
GLOBAL_UNCERTAINTY_ASSIGNED_CONTEXT((#24552))
GLOBAL_UNIT_ASSIGNED_CONTEXT((#24629,#24631,#24632))
REPRESENTATION_CONTEXT('','3D')
) ;
#24628=(
GEOMETRIC_REPRESENTATION_CONTEXT(3)
GLOBAL_UNCERTAINTY_ASSIGNED_CONTEXT((#24580))
GLOBAL_UNIT_ASSIGNED_CONTEXT((#24629,#24631,#24632))
REPRESENTATION_CONTEXT('','3D')
) ;
#24629=(
LENGTH_UNIT()
NAMED_UNIT(*)
SI_UNIT(.CENTI.,.METRE.)
) ;
#24631=(
NAMED_UNIT(*)
PLANE_ANGLE_UNIT()
SI_UNIT($,.RADIAN.)
) ;
#24632=(
NAMED_UNIT(*)
SI_UNIT($,.STERADIAN.)
SOLID_ANGLE_UNIT()
) ;
#24652=SHAPE_DEFINITION_REPRESENTATION(#24699,#24810) ;
#24699=PRODUCT_DEFINITION_SHAPE('',$,#24858) ;
#24810=SHAPE_REPRESENTATION('',(#14495),#24600) ;
#24838=PRODUCT_DEFINITION_CONTEXT('part definition',#24981,'design') ;
#24858=PRODUCT_DEFINITION('EXTERNAL_SPIRAL_RETURN_PIPE',
'EXTERNAL_SPIRAL_RETURN_PIPE',#24905,#24838) ;
#24905=PRODUCT_DEFINITION_FORMATION('',$,#25002) ;
#24981=APPLICATION_CONTEXT(
'Core Data for Automotive Mechanical Design Process') ;
#24982=PRODUCT_CONTEXT('part definition',#24981,'mechanical') ;
#25002=PRODUCT('EXTERNAL_SPIRAL_RETURN_PIPE','EXTERNAL_SPIRAL_RETURN_PIPE',
$,(#24982)) ;
#25037=PRESENTATION_STYLE_ASSIGNMENT((#25047)) ;
#25047=SURFACE_STYLE_USAGE(.BOTH.,#25057) ;
#25057=SURFACE_SIDE_STYLE('',(#25067)) ;
#25067=SURFACE_STYLE_FILL_AREA(#25077) ;
#25077=FILL_AREA_STYLE('Steel - Galvanized (Small)',(#25087)) ;
#25087=FILL_AREA_STYLE_COLOUR('Steel - Galvanized (Small)',#25097) ;
#25097=COLOUR_RGB('Steel - Galvanized (Small)', 0.31764706, 0.68627451, 0.89019608) ;
ENDSEC;
END-ISO-10303-21;
